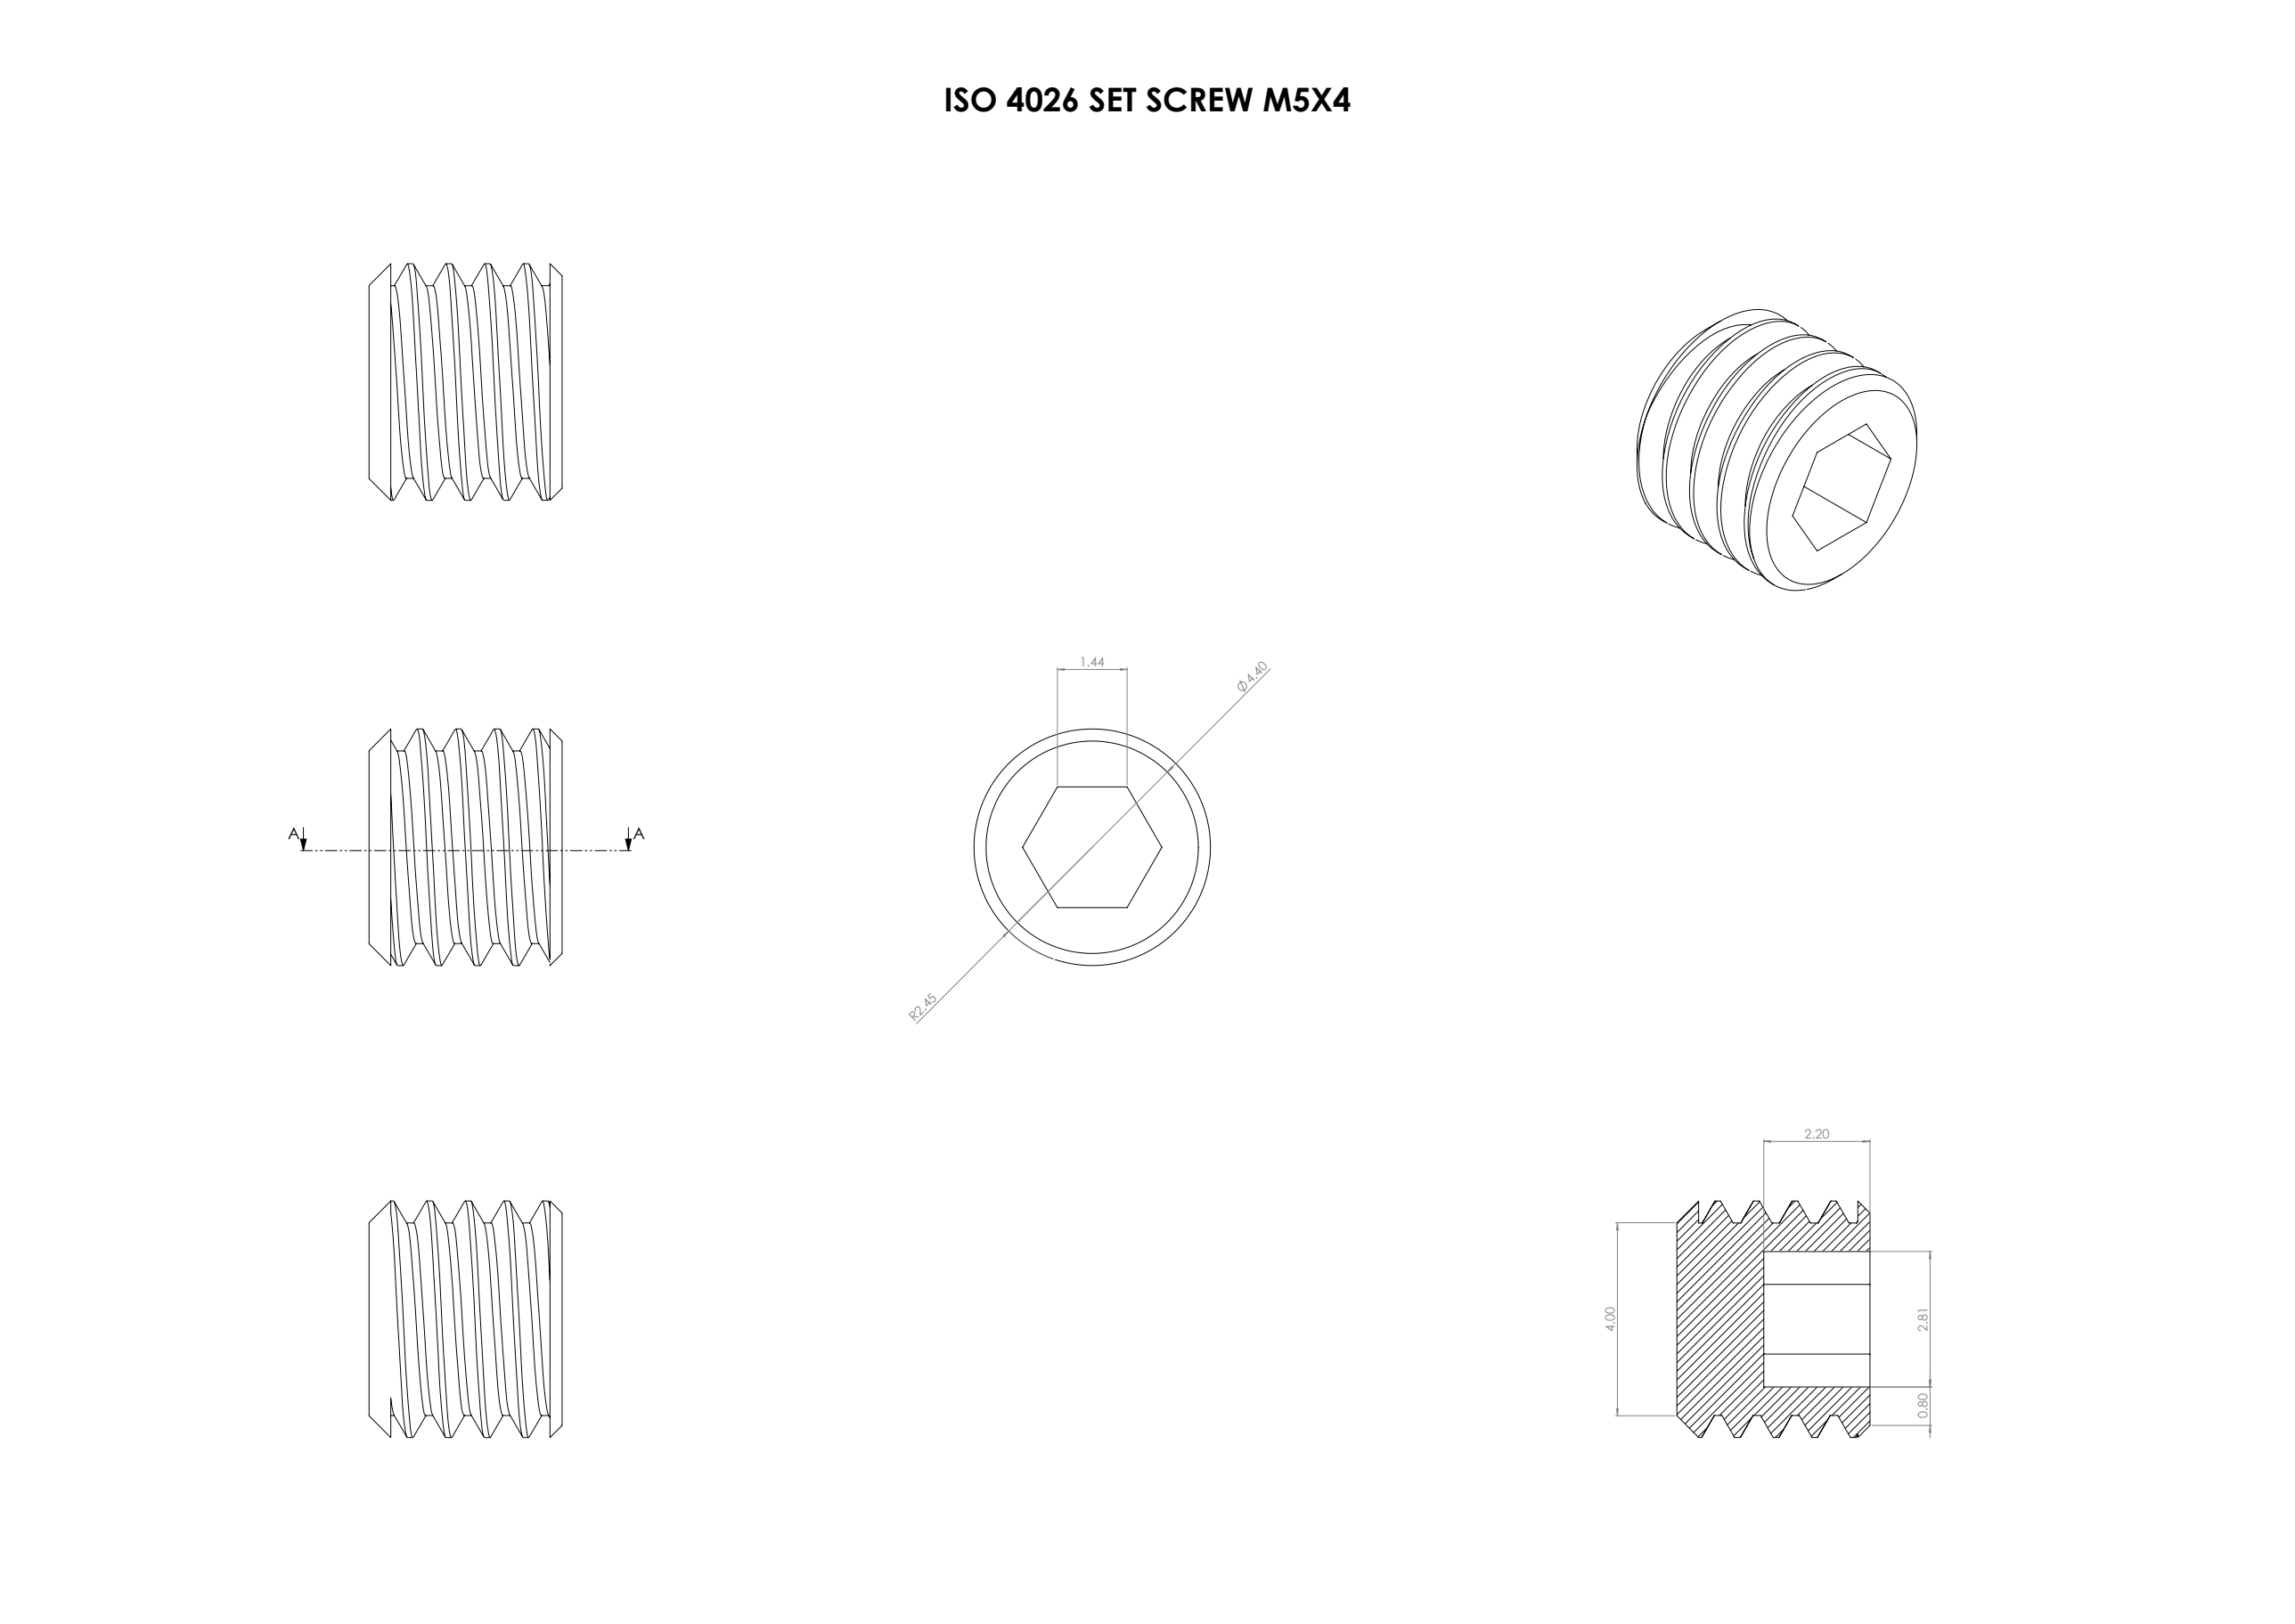
ISO-10303-21;
HEADER;
/* Generated by software containing ST-Developer
 * from STEP Tools, Inc. (www.steptools.com) 
 */

FILE_DESCRIPTION(
/* description */ (''),
/* implementation_level */ '2;1');

FILE_NAME(
/* name */ '11_ISO_4026_Set_Screw_M5x4.step',
/* time_stamp */ '2026-10-21T02:03:06-07:00',
/* author */ (''),
/* organization */ (''),
/* preprocessor_version */ 'ST-DEVELOPER v20.2',
/* originating_system */ 'Autodesk Translation Framework v15.15.0.0',
/* authorisation */ '');

FILE_SCHEMA (('AUTOMOTIVE_DESIGN { 1 0 10303 214 3 1 1 }'));
ENDSEC;

DATA;
#10=MECHANICAL_DESIGN_GEOMETRIC_PRESENTATION_REPRESENTATION('',(#125),#38528);
#87=B_SPLINE_SURFACE_WITH_KNOTS('',3,3,((#35032,#35033,#35034,#35035,#35036,
#35037,#35038,#35039,#35040,#35041,#35042,#35043,#35044,#35045,#35046,#35047,
#35048,#35049,#35050,#35051,#35052,#35053,#35054,#35055,#35056,#35057,#35058,
#35059,#35060,#35061,#35062),(#35063,#35064,#35065,#35066,#35067,#35068,
#35069,#35070,#35071,#35072,#35073,#35074,#35075,#35076,#35077,#35078,#35079,
#35080,#35081,#35082,#35083,#35084,#35085,#35086,#35087,#35088,#35089,#35090,
#35091,#35092,#35093),(#35094,#35095,#35096,#35097,#35098,#35099,#35100,
#35101,#35102,#35103,#35104,#35105,#35106,#35107,#35108,#35109,#35110,#35111,
#35112,#35113,#35114,#35115,#35116,#35117,#35118,#35119,#35120,#35121,#35122,
#35123,#35124),(#35125,#35126,#35127,#35128,#35129,#35130,#35131,#35132,
#35133,#35134,#35135,#35136,#35137,#35138,#35139,#35140,#35141,#35142,#35143,
#35144,#35145,#35146,#35147,#35148,#35149,#35150,#35151,#35152,#35153,#35154,
#35155)),.UNSPECIFIED.,.F.,.F.,.F.,(4,4),(4,1,1,1,1,1,1,1,1,1,1,1,1,1,1,
1,1,1,1,1,1,1,1,1,1,1,1,1,4),(0.,0.0526254770366344),(8.30815772716268,
9.30733212220219,10.3065065172417,11.3056809122812,12.3048553073207,13.3040297023602,
14.3032040973997,15.3023784924392,16.3015528874787,17.3007272825182,18.2999016775577,
19.2990760725973,20.2982504676368,21.2974248626763,22.2965992577158,23.2957736527553,
24.2949480477948,25.2941224428343,26.2932968378738,27.2924712329133,28.2916456279528,
29.2908200229923,30.2899944180318,31.2891688130713,32.2883432081108,33.2875176031503,
34.2866919981899,35.2858663932294,36.2850407882689),.UNSPECIFIED.);
#88=B_SPLINE_SURFACE_WITH_KNOTS('',3,3,((#35379,#35380,#35381,#35382,#35383,
#35384,#35385,#35386,#35387,#35388,#35389,#35390,#35391,#35392,#35393,#35394,
#35395,#35396,#35397,#35398,#35399,#35400,#35401,#35402,#35403,#35404,#35405,
#35406,#35407,#35408,#35409),(#35410,#35411,#35412,#35413,#35414,#35415,
#35416,#35417,#35418,#35419,#35420,#35421,#35422,#35423,#35424,#35425,#35426,
#35427,#35428,#35429,#35430,#35431,#35432,#35433,#35434,#35435,#35436,#35437,
#35438,#35439,#35440),(#35441,#35442,#35443,#35444,#35445,#35446,#35447,
#35448,#35449,#35450,#35451,#35452,#35453,#35454,#35455,#35456,#35457,#35458,
#35459,#35460,#35461,#35462,#35463,#35464,#35465,#35466,#35467,#35468,#35469,
#35470,#35471),(#35472,#35473,#35474,#35475,#35476,#35477,#35478,#35479,
#35480,#35481,#35482,#35483,#35484,#35485,#35486,#35487,#35488,#35489,#35490,
#35491,#35492,#35493,#35494,#35495,#35496,#35497,#35498,#35499,#35500,#35501,
#35502)),.UNSPECIFIED.,.F.,.F.,.F.,(4,4),(4,1,1,1,1,1,1,1,1,1,1,1,1,1,1,
1,1,1,1,1,1,1,1,1,1,1,1,1,4),(0.,0.0526254770366344),(11.6163931973415,
12.615567592381,13.6147419874205,14.61391638246,15.6130907774995,16.612265172539,
17.6114395675785,18.610613962618,19.6097883576575,20.6089627526971,21.6081371477366,
22.6073115427761,23.6064859378156,24.6056603328551,25.6048347278946,26.6040091229341,
27.6031835179736,28.6023579130131,29.6015323080526,30.6007067030921,31.5998810981316,
32.5990554931711,33.5982298882106,34.5974042832501,35.5965786782897,36.5957530733292,
37.5949274683687,38.5941018634082,39.5932762584477),.UNSPECIFIED.);
#101=SHAPE_REPRESENTATION_RELATIONSHIP('SRR','None',#38586,#113);
#113=ADVANCED_BREP_SHAPE_REPRESENTATION('',(#137),#38526);
#125=STYLED_ITEM('',(#38713),#137);
#137=MANIFOLD_SOLID_BREP('Body1',#17082);
#386=CYLINDRICAL_SURFACE('',#18775,2.4505);
#387=CYLINDRICAL_SURFACE('',#18777,2.4505);
#388=CYLINDRICAL_SURFACE('',#18778,2.4505);
#389=CYLINDRICAL_SURFACE('',#18779,2.4505);
#390=CYLINDRICAL_SURFACE('',#18780,1.99475);
#391=CYLINDRICAL_SURFACE('',#18782,1.99475);
#392=CYLINDRICAL_SURFACE('',#18783,1.99475);
#393=CYLINDRICAL_SURFACE('',#18784,1.99475);
#394=CYLINDRICAL_SURFACE('',#18792,1.99475);
#395=CYLINDRICAL_SURFACE('',#18803,2.4505);
#757=B_SPLINE_CURVE_WITH_KNOTS('',3,(#34595,#34596,#34597,#34598,#34599,
#34600,#34601,#34602,#34603,#34604),.UNSPECIFIED.,.F.,.F.,(4,3,3,4),(-4.09157007060746,
-3.99669758015803,-2.99752318511852,-2.06659765062436),.UNSPECIFIED.);
#758=B_SPLINE_CURVE_WITH_KNOTS('',3,(#34607,#34608,#34609,#34610,#34611,
#34612,#34613),.UNSPECIFIED.,.F.,.F.,(4,3,4),(0.,0.999174395039508,1.11662023360669),
 .UNSPECIFIED.);
#759=B_SPLINE_CURVE_WITH_KNOTS('',3,(#34618,#34619,#34620,#34621,#34622,
#34623,#34624,#34625,#34626,#34627,#34628,#34629,#34630,#34631,#34632,#34633,
#34634,#34635,#34636,#34637,#34638,#34639),.UNSPECIFIED.,.F.,.F.,(4,3,3,
3,3,3,3,4),(-10.3747553777871,-9.99174395039507,-8.99256955535556,-7.99339516031606,
-6.99422076527655,-5.99504637023704,-4.99587197519754,-4.09157007060746),
 .UNSPECIFIED.);
#760=B_SPLINE_CURVE_WITH_KNOTS('',3,(#34640,#34641,#34642,#34643,#34644,
#34645,#34646,#34647,#34648,#34649,#34650,#34651,#34652,#34653,#34654,#34655,
#34656,#34657,#34658,#34659,#34660,#34661),.UNSPECIFIED.,.F.,.F.,(4,3,3,
3,3,3,3,4),(1.11662023360669,1.99834879007901,2.99752318511852,3.99669758015803,
4.99587197519753,5.99504637023704,6.99422076527654,7.39980554078627),
 .UNSPECIFIED.);
#761=B_SPLINE_CURVE_WITH_KNOTS('',3,(#34666,#34667,#34668,#34669,#34670,
#34671,#34672,#34673,#34674,#34675,#34676,#34677,#34678,#34679,#34680,#34681,
#34682,#34683,#34684,#34685,#34686,#34687),.UNSPECIFIED.,.F.,.F.,(4,3,3,
3,3,3,3,4),(-16.6579406849666,-15.9867903206321,-14.9876159255926,-13.9884415305531,
-12.9892671355136,-11.9900927404741,-10.9909183454346,-10.3747553777871),
 .UNSPECIFIED.);
#762=B_SPLINE_CURVE_WITH_KNOTS('',3,(#34688,#34689,#34690,#34691,#34692,
#34693,#34694,#34695,#34696,#34697,#34698,#34699,#34700,#34701,#34702,#34703,
#34704,#34705,#34706,#34707,#34708,#34709),.UNSPECIFIED.,.F.,.F.,(4,3,3,
3,3,3,3,4),(7.39980554078627,7.99339516031605,8.99256955535556,9.99174395039507,
10.9909183454346,11.9900927404741,12.9892671355136,13.6829908479659),
 .UNSPECIFIED.);
#763=B_SPLINE_CURVE_WITH_KNOTS('',3,(#34714,#34715,#34716,#34717,#34718,
#34719,#34720,#34721,#34722,#34723,#34724,#34725,#34726,#34727,#34728,#34729,
#34730,#34731,#34732,#34733,#34734,#34735),.UNSPECIFIED.,.F.,.F.,(4,3,3,
3,3,3,3,4),(-22.9411259921462,-21.9818366908691,-20.9826622958296,-19.9834879007901,
-18.9843135057506,-17.9851391107111,-16.9859647156716,-16.6579406849666),
 .UNSPECIFIED.);
#764=B_SPLINE_CURVE_WITH_KNOTS('',3,(#34736,#34737,#34738,#34739,#34740,
#34741,#34742,#34743,#34744,#34745,#34746,#34747,#34748,#34749,#34750,#34751,
#34752,#34753,#34754,#34755,#34756,#34757),.UNSPECIFIED.,.F.,.F.,(4,3,3,
3,3,3,3,4),(13.6829908479659,13.9884415305531,14.9876159255926,15.9867903206321,
16.9859647156716,17.9851391107111,18.9843135057506,19.9661761551454),
 .UNSPECIFIED.);
#765=B_SPLINE_CURVE_WITH_KNOTS('',3,(#34763,#34764,#34765,#34766,#34767,
#34768,#34769),.UNSPECIFIED.,.F.,.F.,(4,1,1,1,4),(34.5575191894877,34.5974042832501,
35.5965786782897,36.5957530733292,37.5266786078233),.UNSPECIFIED.);
#766=B_SPLINE_CURVE_WITH_KNOTS('',3,(#34772,#34773,#34774,#34775,#34776),
 .UNSPECIFIED.,.F.,.F.,(4,1,4),(34.5575191894877,35.2858663932294,36.2850407882689),
 .UNSPECIFIED.);
#767=B_SPLINE_CURVE_WITH_KNOTS('',3,(#34781,#34782,#34783,#34784,#34785,
#34786,#34787,#34788,#34789,#34790),.UNSPECIFIED.,.F.,.F.,(4,1,1,1,1,1,
1,4),(28.2743338823081,28.6023579130131,29.6015323080526,30.6007067030921,
31.5998810981316,32.5990554931711,33.5982298882106,34.5575191894877),
 .UNSPECIFIED.);
#768=B_SPLINE_CURVE_WITH_KNOTS('',3,(#34791,#34792,#34793,#34794,#34795,
#34796,#34797,#34798,#34799,#34800,#34801),.UNSPECIFIED.,.F.,.F.,(4,1,1,
1,1,1,1,1,4),(28.2743338823081,28.2916456279528,29.2908200229923,30.2899944180318,
31.2891688130713,32.2883432081108,33.2875176031503,34.2866919981899,34.5575191894877),
 .UNSPECIFIED.);
#769=B_SPLINE_CURVE_WITH_KNOTS('',3,(#34806,#34807,#34808,#34809,#34810,
#34811,#34812,#34813,#34814,#34815),.UNSPECIFIED.,.F.,.F.,(4,1,1,1,1,1,
1,4),(21.9911485751285,22.6073115427761,23.6064859378156,24.6056603328551,
25.6048347278946,26.6040091229341,27.6031835179736,28.2743338823081),
 .UNSPECIFIED.);
#770=B_SPLINE_CURVE_WITH_KNOTS('',3,(#34816,#34817,#34818,#34819,#34820,
#34821,#34822,#34823,#34824,#34825),.UNSPECIFIED.,.F.,.F.,(4,1,1,1,1,1,
1,4),(21.9911485751285,22.2965992577158,23.2957736527553,24.2949480477948,
25.2941224428343,26.2932968378738,27.2924712329133,28.2743338823081),
 .UNSPECIFIED.);
#771=B_SPLINE_CURVE_WITH_KNOTS('',3,(#34830,#34831,#34832,#34833,#34834,
#34835,#34836,#34837,#34838,#34839),.UNSPECIFIED.,.F.,.F.,(4,1,1,1,1,1,
1,4),(15.707963267949,16.612265172539,17.6114395675785,18.610613962618,
19.6097883576575,20.6089627526971,21.6081371477366,21.9911485751285),
 .UNSPECIFIED.);
#772=B_SPLINE_CURVE_WITH_KNOTS('',3,(#34840,#34841,#34842,#34843,#34844,
#34845,#34846,#34847,#34848,#34849),.UNSPECIFIED.,.F.,.F.,(4,1,1,1,1,1,
1,4),(15.707963267949,16.3015528874787,17.3007272825182,18.2999016775577,
19.2990760725973,20.2982504676368,21.2974248626763,21.9911485751285),
 .UNSPECIFIED.);
#773=B_SPLINE_CURVE_WITH_KNOTS('',3,(#34852,#34853,#34854,#34855,#34856,
#34857,#34858,#34859,#34860,#34861,#34862,#34863,#34864,#34865,#34866,#34867,
#34868,#34869,#34870,#34871,#34872,#34873,#34874,#34875,#34876,#34877,#34878,
#34879,#34880,#34881,#34882,#34883,#34884,#34885,#34886,#34887,#34888,#34889,
#34890,#34891,#34892,#34893,#34894,#34895,#34896,#34897,#34898,#34899,#34900,
#34901,#34902,#34903,#34904,#34905,#34906,#34907,#34908,#34909,#34910,#34911,
#34912,#34913,#34914,#34915,#34916,#34917,#34918,#34919,#34920,#34921,#34922,
#34923,#34924,#34925,#34926,#34927,#34928,#34929,#34930,#34931,#34932,#34933,
#34934,#34935,#34936,#34937,#34938,#34939),.UNSPECIFIED.,.F.,.F.,(4,3,3,
3,3,3,3,3,3,3,3,3,3,3,3,3,3,3,3,3,3,3,3,3,3,3,3,3,3,4),(-0.463803050843695,
-0.449990761124198,-0.428296524385296,-0.416270113415759,-0.41034182721078,
-0.406031993683804,-0.383353142504459,-0.364918243300489,-0.357623436893478,
-0.352445440792161,-0.329117850494041,-0.305348418252453,-0.287979800907514,
-0.27495333789881,-0.271003592095896,-0.246574718000476,-0.235873948872699,
-0.212294861299806,-0.188221669997877,-0.184247659311273,-0.180472049728776,
-0.156013909098849,-0.131078945975368,-0.105968578777427,-0.0960005902951454,
-0.0910052533817002,-0.0652636023140419,-0.03948256399711,-0.0142485222596106,
0.),.UNSPECIFIED.);
#774=B_SPLINE_CURVE_WITH_KNOTS('',3,(#34944,#34945,#34946,#34947,#34948,
#34949,#34950,#34951,#34952,#34953,#34954,#34955,#34956,#34957,#34958,#34959,
#34960,#34961,#34962,#34963,#34964,#34965,#34966,#34967,#34968,#34969,#34970,
#34971,#34972,#34973,#34974,#34975,#34976,#34977,#34978,#34979,#34980,#34981,
#34982,#34983,#34984,#34985,#34986,#34987,#34988,#34989,#34990,#34991,#34992,
#34993,#34994,#34995,#34996,#34997,#34998,#34999,#35000,#35001,#35002,#35003,
#35004,#35005,#35006,#35007,#35008,#35009,#35010,#35011,#35012,#35013,#35014,
#35015,#35016,#35017,#35018,#35019,#35020,#35021,#35022,#35023,#35024,#35025,
#35026,#35027,#35028,#35029,#35030,#35031),.UNSPECIFIED.,.F.,.F.,(4,3,3,
3,3,3,3,3,3,3,3,3,3,3,3,3,3,3,3,3,3,3,3,3,3,3,3,3,3,4),(-0.46178896489977,
-0.445096409523187,-0.41948010739612,-0.406506945826406,-0.398412550454382,
-0.393270804127913,-0.367882741380425,-0.348386088992959,-0.338710078205615,
-0.332907547801024,-0.308142244019199,-0.283899773513071,-0.26018963968495,
-0.251870459427571,-0.247081329031836,-0.243331119007966,-0.219855106139638,
-0.211909522280695,-0.187951737144655,-0.164457770001573,-0.15868347025795,
-0.135324913286723,-0.111987831540051,-0.0890431146252489,-0.0803312568299254,
-0.0766174929132729,-0.0541552161857382,-0.0320577725876878,-0.0106683587118627,
0.),.UNSPECIFIED.);
#775=B_SPLINE_CURVE_WITH_KNOTS('',3,(#35156,#35157,#35158,#35159,#35160,
#35161,#35162,#35163,#35164,#35165,#35166,#35167,#35168,#35169,#35170,#35171,
#35172,#35173,#35174,#35175,#35176,#35177),.UNSPECIFIED.,.F.,.F.,(4,3,3,
3,3,3,3,4),(19.9661761551454,19.9834879007901,20.9826622958296,21.9818366908691,
22.9810110859087,23.9801854809482,24.9793598759877,25.9102854104818),
 .UNSPECIFIED.);
#776=B_SPLINE_CURVE_WITH_KNOTS('',3,(#35179,#35180,#35181,#35182,#35183,
#35184,#35185,#35186,#35187,#35188,#35189,#35190,#35191,#35192,#35193,#35194,
#35195,#35196,#35197,#35198,#35199,#35200,#35201,#35202,#35203,#35204,#35205,
#35206,#35207,#35208,#35209,#35210,#35211,#35212,#35213,#35214,#35215,#35216,
#35217,#35218,#35219,#35220,#35221,#35222,#35223,#35224,#35225,#35226,#35227,
#35228,#35229,#35230,#35231,#35232,#35233,#35234,#35235,#35236,#35237,#35238,
#35239,#35240,#35241,#35242,#35243,#35244,#35245,#35246,#35247,#35248,#35249,
#35250,#35251,#35252,#35253,#35254,#35255,#35256,#35257,#35258,#35259,#35260,
#35261,#35262,#35263,#35264,#35265,#35266),.UNSPECIFIED.,.F.,.F.,(4,3,3,
3,3,3,3,3,3,3,3,3,3,3,3,3,3,3,3,3,3,3,3,3,3,3,3,3,3,4),(-0.463803050843709,
-0.449990761124214,-0.428296490111524,-0.416270081284097,-0.410341690806036,
-0.406031962003142,-0.383353089621238,-0.364918197027671,-0.357623306842884,
-0.35244540774759,-0.329117799946646,-0.305348369315656,-0.287979764204916,
-0.274953310371862,-0.271003565635767,-0.246574693089584,-0.235873948872699,
-0.21229484773092,-0.188221640039157,-0.184247642913191,-0.180472048117772,
-0.15601389132531,-0.131078912920519,-0.105968544178087,-0.096000611432122,
-0.0910052576643347,-0.0652635971708748,-0.0394825672375708,-0.014248568646013,
0.),.UNSPECIFIED.);
#777=B_SPLINE_CURVE_WITH_KNOTS('',3,(#35267,#35268,#35269,#35270,#35271,
#35272,#35273,#35274,#35275),.UNSPECIFIED.,.F.,.F.,(4,1,1,1,1,1,4),(10.374755377787,
11.3056809122812,12.3048553073207,13.3040297023602,14.3032040973997,15.3023784924392,
15.707963267949),.UNSPECIFIED.);
#778=B_SPLINE_CURVE_WITH_KNOTS('',3,(#35281,#35282,#35283,#35284,#35285,
#35286,#35287,#35288,#35289,#35290,#35291,#35292,#35293,#35294,#35295,#35296,
#35297,#35298,#35299,#35300,#35301,#35302,#35303,#35304,#35305,#35306,#35307,
#35308,#35309,#35310,#35311,#35312,#35313,#35314,#35315,#35316,#35317,#35318,
#35319,#35320,#35321,#35322,#35323,#35324,#35325,#35326,#35327,#35328,#35329,
#35330,#35331,#35332,#35333,#35334,#35335,#35336,#35337,#35338,#35339,#35340,
#35341,#35342,#35343,#35344,#35345,#35346,#35347,#35348,#35349,#35350,#35351,
#35352,#35353,#35354,#35355,#35356,#35357,#35358,#35359,#35360,#35361,#35362,
#35363,#35364,#35365,#35366,#35367,#35368),.UNSPECIFIED.,.F.,.F.,(4,3,3,
3,3,3,3,3,3,3,3,3,3,3,3,3,3,3,3,3,3,3,3,3,3,3,3,3,3,4),(-0.461788964899768,
-0.445096409523188,-0.419480109352795,-0.406506947660789,-0.398412571668129,
-0.393270813953603,-0.367882751783358,-0.348386098095525,-0.338710098423989,
-0.332907549361998,-0.308142248257406,-0.283899804164729,-0.260189710156508,
-0.251870630384198,-0.247081550599562,-0.243331158606442,-0.219855173637982,
-0.211909522280694,-0.187951756384898,-0.164457786836786,-0.158683460701996,
-0.135324913663822,-0.111987815902327,-0.0890430596778552,-0.0803312466615788,
-0.0766174883386559,-0.0541551823514923,-0.0320576942341872,-0.0106682241746107,
0.),.UNSPECIFIED.);
#779=B_SPLINE_CURVE_WITH_KNOTS('',3,(#35371,#35372,#35373,#35374,#35375,
#35376,#35377,#35378),.UNSPECIFIED.,.F.,.F.,(4,1,1,1,1,4),(11.6163931973415,
12.615567592381,13.6147419874205,14.61391638246,15.6130907774995,15.707963267949),
 .UNSPECIFIED.);
#780=B_SPLINE_CURVE_WITH_KNOTS('',3,(#35503,#35504,#35505,#35506,#35507,
#35508,#35509,#35510,#35511,#35512,#35513,#35514,#35515,#35516,#35517,#35518,
#35519,#35520,#35521),.UNSPECIFIED.,.F.,.F.,(4,3,3,3,3,3,4),(-27.9768830611062,
-26.9777086660667,-25.9785342710272,-24.9793598759877,-23.9801854809482,
-22.9810110859087,-22.9411259921462),.UNSPECIFIED.);
#1046=CONICAL_SURFACE('',#18802,2.25,0.785398163397448);
#1047=CONICAL_SURFACE('',#18805,2.35,0.785398163397447);
#1475=FACE_BOUND('',#4158,.T.);
#2199=CIRCLE('',#18776,2.4505);
#2200=CIRCLE('',#18781,1.99475);
#2201=CIRCLE('',#18786,2.4505);
#2202=CIRCLE('',#18787,2.4505);
#2203=CIRCLE('',#18789,2.4505);
#2204=CIRCLE('',#18790,2.4505);
#2205=CIRCLE('',#18791,1.99475);
#2206=CIRCLE('',#18801,2.);
#2207=CIRCLE('',#18804,2.4505);
#2208=CIRCLE('',#18806,2.2);
#3107=FACE_OUTER_BOUND('',#4133,.T.);
#3108=FACE_OUTER_BOUND('',#4134,.T.);
#3109=FACE_OUTER_BOUND('',#4135,.T.);
#3110=FACE_OUTER_BOUND('',#4136,.T.);
#3111=FACE_OUTER_BOUND('',#4137,.T.);
#3112=FACE_OUTER_BOUND('',#4138,.T.);
#3113=FACE_OUTER_BOUND('',#4139,.T.);
#3114=FACE_OUTER_BOUND('',#4140,.T.);
#3115=FACE_OUTER_BOUND('',#4141,.T.);
#3116=FACE_OUTER_BOUND('',#4142,.T.);
#3117=FACE_OUTER_BOUND('',#4143,.T.);
#3118=FACE_OUTER_BOUND('',#4144,.T.);
#3119=FACE_OUTER_BOUND('',#4145,.T.);
#3120=FACE_OUTER_BOUND('',#4146,.T.);
#3121=FACE_OUTER_BOUND('',#4147,.T.);
#3122=FACE_OUTER_BOUND('',#4148,.T.);
#3123=FACE_OUTER_BOUND('',#4149,.T.);
#3124=FACE_OUTER_BOUND('',#4150,.T.);
#3125=FACE_OUTER_BOUND('',#4151,.T.);
#3126=FACE_OUTER_BOUND('',#4152,.T.);
#3127=FACE_OUTER_BOUND('',#4153,.T.);
#3128=FACE_OUTER_BOUND('',#4154,.T.);
#3129=FACE_OUTER_BOUND('',#4155,.T.);
#3130=FACE_OUTER_BOUND('',#4156,.T.);
#3131=FACE_OUTER_BOUND('',#4157,.T.);
#4133=EDGE_LOOP('',(#14731,#14732,#14733,#14734));
#4134=EDGE_LOOP('',(#14735,#14736,#14737,#14738));
#4135=EDGE_LOOP('',(#14739,#14740,#14741,#14742));
#4136=EDGE_LOOP('',(#14743,#14744,#14745,#14746));
#4137=EDGE_LOOP('',(#14747,#14748,#14749,#14750));
#4138=EDGE_LOOP('',(#14751,#14752,#14753,#14754));
#4139=EDGE_LOOP('',(#14755,#14756,#14757,#14758));
#4140=EDGE_LOOP('',(#14759,#14760,#14761,#14762));
#4141=EDGE_LOOP('',(#14763,#14764,#14765,#14766,#14767));
#4142=EDGE_LOOP('',(#14768,#14769,#14770,#14771,#14772,#14773,#14774,#14775,
#14776,#14777,#14778,#14779));
#4143=EDGE_LOOP('',(#14780,#14781,#14782,#14783,#14784));
#4144=EDGE_LOOP('',(#14785,#14786,#14787,#14788));
#4145=EDGE_LOOP('',(#14789,#14790,#14791,#14792,#14793,#14794,#14795,#14796,
#14797,#14798,#14799,#14800));
#4146=EDGE_LOOP('',(#14801,#14802,#14803,#14804));
#4147=EDGE_LOOP('',(#14805,#14806,#14807,#14808));
#4148=EDGE_LOOP('',(#14809,#14810,#14811,#14812));
#4149=EDGE_LOOP('',(#14813,#14814,#14815,#14816));
#4150=EDGE_LOOP('',(#14817,#14818,#14819,#14820));
#4151=EDGE_LOOP('',(#14821,#14822,#14823,#14824));
#4152=EDGE_LOOP('',(#14825,#14826,#14827,#14828,#14829,#14830));
#4153=EDGE_LOOP('',(#14831));
#4154=EDGE_LOOP('',(#14832,#14833,#14834,#14835,#14836,#14837));
#4155=EDGE_LOOP('',(#14838,#14839,#14840,#14841));
#4156=EDGE_LOOP('',(#14842,#14843,#14844,#14845,#14846,#14847));
#4157=EDGE_LOOP('',(#14848));
#4158=EDGE_LOOP('',(#14849,#14850,#14851,#14852,#14853,#14854));
#5055=LINE('',#34593,#6030);
#5056=LINE('',#34617,#6031);
#5057=LINE('',#34665,#6032);
#5058=LINE('',#34713,#6033);
#5059=LINE('',#34761,#6034);
#5060=LINE('',#34780,#6035);
#5061=LINE('',#34805,#6036);
#5062=LINE('',#34829,#6037);
#5063=LINE('',#35525,#6038);
#5064=LINE('',#35527,#6039);
#5065=LINE('',#35529,#6040);
#5066=LINE('',#35530,#6041);
#5067=LINE('',#35533,#6042);
#5068=LINE('',#35535,#6043);
#5069=LINE('',#35536,#6044);
#5070=LINE('',#35539,#6045);
#5071=LINE('',#35541,#6046);
#5072=LINE('',#35542,#6047);
#5073=LINE('',#35545,#6048);
#5074=LINE('',#35547,#6049);
#5075=LINE('',#35548,#6050);
#5076=LINE('',#35551,#6051);
#5077=LINE('',#35553,#6052);
#5078=LINE('',#35554,#6053);
#5079=LINE('',#35556,#6054);
#5080=LINE('',#35557,#6055);
#5081=LINE('',#35563,#6056);
#5082=LINE('',#35569,#6057);
#6030=VECTOR('',#22907,2.5);
#6031=VECTOR('',#22912,2.5);
#6032=VECTOR('',#22915,2.5);
#6033=VECTOR('',#22918,2.5);
#6034=VECTOR('',#22921,1.99475);
#6035=VECTOR('',#22926,1.99475);
#6036=VECTOR('',#22929,1.99475);
#6037=VECTOR('',#22932,1.99475);
#6038=VECTOR('',#22951,10.);
#6039=VECTOR('',#22952,10.);
#6040=VECTOR('',#22953,10.);
#6041=VECTOR('',#22954,10.);
#6042=VECTOR('',#22957,10.);
#6043=VECTOR('',#22958,10.);
#6044=VECTOR('',#22959,10.);
#6045=VECTOR('',#22962,10.);
#6046=VECTOR('',#22963,10.);
#6047=VECTOR('',#22964,10.);
#6048=VECTOR('',#22967,10.);
#6049=VECTOR('',#22968,10.);
#6050=VECTOR('',#22969,10.);
#6051=VECTOR('',#22972,10.);
#6052=VECTOR('',#22973,10.);
#6053=VECTOR('',#22974,10.);
#6054=VECTOR('',#22977,10.);
#6055=VECTOR('',#22978,10.);
#6056=VECTOR('',#22987,2.25);
#6057=VECTOR('',#22996,2.35);
#7589=VERTEX_POINT('',#34591);
#7590=VERTEX_POINT('',#34592);
#7591=VERTEX_POINT('',#34594);
#7592=VERTEX_POINT('',#34605);
#7593=VERTEX_POINT('',#34615);
#7594=VERTEX_POINT('',#34616);
#7595=VERTEX_POINT('',#34663);
#7596=VERTEX_POINT('',#34664);
#7597=VERTEX_POINT('',#34711);
#7598=VERTEX_POINT('',#34712);
#7599=VERTEX_POINT('',#34759);
#7600=VERTEX_POINT('',#34760);
#7601=VERTEX_POINT('',#34762);
#7602=VERTEX_POINT('',#34770);
#7603=VERTEX_POINT('',#34778);
#7604=VERTEX_POINT('',#34779);
#7605=VERTEX_POINT('',#34803);
#7606=VERTEX_POINT('',#34804);
#7607=VERTEX_POINT('',#34827);
#7608=VERTEX_POINT('',#34828);
#7609=VERTEX_POINT('',#34851);
#7610=VERTEX_POINT('',#34940);
#7611=VERTEX_POINT('',#34942);
#7612=VERTEX_POINT('',#35178);
#7613=VERTEX_POINT('',#35277);
#7614=VERTEX_POINT('',#35280);
#7615=VERTEX_POINT('',#35523);
#7616=VERTEX_POINT('',#35524);
#7617=VERTEX_POINT('',#35526);
#7618=VERTEX_POINT('',#35528);
#7619=VERTEX_POINT('',#35532);
#7620=VERTEX_POINT('',#35534);
#7621=VERTEX_POINT('',#35538);
#7622=VERTEX_POINT('',#35540);
#7623=VERTEX_POINT('',#35544);
#7624=VERTEX_POINT('',#35546);
#7625=VERTEX_POINT('',#35550);
#7626=VERTEX_POINT('',#35552);
#7627=VERTEX_POINT('',#35560);
#7628=VERTEX_POINT('',#35567);
#10017=EDGE_CURVE('',#7589,#7590,#5055,.T.);
#10018=EDGE_CURVE('',#7589,#7591,#757,.T.);
#10019=EDGE_CURVE('',#7591,#7592,#2199,.T.);
#10020=EDGE_CURVE('',#7592,#7590,#758,.T.);
#10021=EDGE_CURVE('',#7593,#7594,#5056,.T.);
#10022=EDGE_CURVE('',#7593,#7589,#759,.T.);
#10023=EDGE_CURVE('',#7590,#7594,#760,.T.);
#10024=EDGE_CURVE('',#7595,#7596,#5057,.T.);
#10025=EDGE_CURVE('',#7595,#7593,#761,.T.);
#10026=EDGE_CURVE('',#7594,#7596,#762,.T.);
#10027=EDGE_CURVE('',#7597,#7598,#5058,.T.);
#10028=EDGE_CURVE('',#7597,#7595,#763,.T.);
#10029=EDGE_CURVE('',#7596,#7598,#764,.T.);
#10030=EDGE_CURVE('',#7599,#7600,#5059,.T.);
#10031=EDGE_CURVE('',#7599,#7601,#765,.T.);
#10032=EDGE_CURVE('',#7602,#7601,#2200,.T.);
#10033=EDGE_CURVE('',#7600,#7602,#766,.T.);
#10034=EDGE_CURVE('',#7603,#7604,#5060,.T.);
#10035=EDGE_CURVE('',#7603,#7599,#767,.T.);
#10036=EDGE_CURVE('',#7604,#7600,#768,.T.);
#10037=EDGE_CURVE('',#7605,#7606,#5061,.T.);
#10038=EDGE_CURVE('',#7605,#7603,#769,.T.);
#10039=EDGE_CURVE('',#7606,#7604,#770,.T.);
#10040=EDGE_CURVE('',#7607,#7608,#5062,.T.);
#10041=EDGE_CURVE('',#7607,#7605,#771,.T.);
#10042=EDGE_CURVE('',#7608,#7606,#772,.T.);
#10043=EDGE_CURVE('',#7601,#7609,#773,.T.);
#10044=EDGE_CURVE('',#7610,#7609,#2201,.F.);
#10045=EDGE_CURVE('',#7611,#7610,#2202,.F.);
#10046=EDGE_CURVE('',#7611,#7602,#774,.T.);
#10047=EDGE_CURVE('',#7598,#7611,#775,.T.);
#10048=EDGE_CURVE('',#7612,#7592,#776,.T.);
#10049=EDGE_CURVE('',#7612,#7608,#777,.T.);
#10050=EDGE_CURVE('',#7592,#7613,#2203,.T.);
#10051=EDGE_CURVE('',#7613,#7591,#2204,.T.);
#10052=EDGE_CURVE('',#7591,#7614,#778,.T.);
#10053=EDGE_CURVE('',#7614,#7612,#2205,.T.);
#10054=EDGE_CURVE('',#7614,#7607,#779,.T.);
#10055=EDGE_CURVE('',#7609,#7597,#780,.T.);
#10056=EDGE_CURVE('',#7615,#7616,#5063,.T.);
#10057=EDGE_CURVE('',#7615,#7617,#5064,.T.);
#10058=EDGE_CURVE('',#7617,#7618,#5065,.T.);
#10059=EDGE_CURVE('',#7616,#7618,#5066,.T.);
#10060=EDGE_CURVE('',#7619,#7615,#5067,.T.);
#10061=EDGE_CURVE('',#7619,#7620,#5068,.T.);
#10062=EDGE_CURVE('',#7620,#7617,#5069,.T.);
#10063=EDGE_CURVE('',#7621,#7619,#5070,.T.);
#10064=EDGE_CURVE('',#7621,#7622,#5071,.T.);
#10065=EDGE_CURVE('',#7622,#7620,#5072,.T.);
#10066=EDGE_CURVE('',#7623,#7621,#5073,.T.);
#10067=EDGE_CURVE('',#7623,#7624,#5074,.T.);
#10068=EDGE_CURVE('',#7624,#7622,#5075,.T.);
#10069=EDGE_CURVE('',#7625,#7623,#5076,.T.);
#10070=EDGE_CURVE('',#7625,#7626,#5077,.T.);
#10071=EDGE_CURVE('',#7626,#7624,#5078,.T.);
#10072=EDGE_CURVE('',#7616,#7625,#5079,.T.);
#10073=EDGE_CURVE('',#7618,#7626,#5080,.T.);
#10074=EDGE_CURVE('',#7627,#7627,#2206,.T.);
#10075=EDGE_CURVE('',#7613,#7627,#5081,.T.);
#10076=EDGE_CURVE('',#7609,#7611,#2207,.F.);
#10077=EDGE_CURVE('',#7628,#7628,#2208,.T.);
#10078=EDGE_CURVE('',#7628,#7610,#5082,.T.);
#14731=ORIENTED_EDGE('',*,*,#10017,.F.);
#14732=ORIENTED_EDGE('',*,*,#10018,.T.);
#14733=ORIENTED_EDGE('',*,*,#10019,.T.);
#14734=ORIENTED_EDGE('',*,*,#10020,.T.);
#14735=ORIENTED_EDGE('',*,*,#10021,.F.);
#14736=ORIENTED_EDGE('',*,*,#10022,.T.);
#14737=ORIENTED_EDGE('',*,*,#10017,.T.);
#14738=ORIENTED_EDGE('',*,*,#10023,.T.);
#14739=ORIENTED_EDGE('',*,*,#10024,.F.);
#14740=ORIENTED_EDGE('',*,*,#10025,.T.);
#14741=ORIENTED_EDGE('',*,*,#10021,.T.);
#14742=ORIENTED_EDGE('',*,*,#10026,.T.);
#14743=ORIENTED_EDGE('',*,*,#10027,.F.);
#14744=ORIENTED_EDGE('',*,*,#10028,.T.);
#14745=ORIENTED_EDGE('',*,*,#10024,.T.);
#14746=ORIENTED_EDGE('',*,*,#10029,.T.);
#14747=ORIENTED_EDGE('',*,*,#10030,.F.);
#14748=ORIENTED_EDGE('',*,*,#10031,.T.);
#14749=ORIENTED_EDGE('',*,*,#10032,.F.);
#14750=ORIENTED_EDGE('',*,*,#10033,.F.);
#14751=ORIENTED_EDGE('',*,*,#10034,.F.);
#14752=ORIENTED_EDGE('',*,*,#10035,.T.);
#14753=ORIENTED_EDGE('',*,*,#10030,.T.);
#14754=ORIENTED_EDGE('',*,*,#10036,.F.);
#14755=ORIENTED_EDGE('',*,*,#10037,.F.);
#14756=ORIENTED_EDGE('',*,*,#10038,.T.);
#14757=ORIENTED_EDGE('',*,*,#10034,.T.);
#14758=ORIENTED_EDGE('',*,*,#10039,.F.);
#14759=ORIENTED_EDGE('',*,*,#10040,.F.);
#14760=ORIENTED_EDGE('',*,*,#10041,.T.);
#14761=ORIENTED_EDGE('',*,*,#10037,.T.);
#14762=ORIENTED_EDGE('',*,*,#10042,.F.);
#14763=ORIENTED_EDGE('',*,*,#10032,.T.);
#14764=ORIENTED_EDGE('',*,*,#10043,.T.);
#14765=ORIENTED_EDGE('',*,*,#10044,.F.);
#14766=ORIENTED_EDGE('',*,*,#10045,.F.);
#14767=ORIENTED_EDGE('',*,*,#10046,.T.);
#14768=ORIENTED_EDGE('',*,*,#10046,.F.);
#14769=ORIENTED_EDGE('',*,*,#10047,.F.);
#14770=ORIENTED_EDGE('',*,*,#10029,.F.);
#14771=ORIENTED_EDGE('',*,*,#10026,.F.);
#14772=ORIENTED_EDGE('',*,*,#10023,.F.);
#14773=ORIENTED_EDGE('',*,*,#10020,.F.);
#14774=ORIENTED_EDGE('',*,*,#10048,.F.);
#14775=ORIENTED_EDGE('',*,*,#10049,.T.);
#14776=ORIENTED_EDGE('',*,*,#10042,.T.);
#14777=ORIENTED_EDGE('',*,*,#10039,.T.);
#14778=ORIENTED_EDGE('',*,*,#10036,.T.);
#14779=ORIENTED_EDGE('',*,*,#10033,.T.);
#14780=ORIENTED_EDGE('',*,*,#10050,.T.);
#14781=ORIENTED_EDGE('',*,*,#10051,.T.);
#14782=ORIENTED_EDGE('',*,*,#10052,.T.);
#14783=ORIENTED_EDGE('',*,*,#10053,.T.);
#14784=ORIENTED_EDGE('',*,*,#10048,.T.);
#14785=ORIENTED_EDGE('',*,*,#10040,.T.);
#14786=ORIENTED_EDGE('',*,*,#10049,.F.);
#14787=ORIENTED_EDGE('',*,*,#10053,.F.);
#14788=ORIENTED_EDGE('',*,*,#10054,.T.);
#14789=ORIENTED_EDGE('',*,*,#10043,.F.);
#14790=ORIENTED_EDGE('',*,*,#10031,.F.);
#14791=ORIENTED_EDGE('',*,*,#10035,.F.);
#14792=ORIENTED_EDGE('',*,*,#10038,.F.);
#14793=ORIENTED_EDGE('',*,*,#10041,.F.);
#14794=ORIENTED_EDGE('',*,*,#10054,.F.);
#14795=ORIENTED_EDGE('',*,*,#10052,.F.);
#14796=ORIENTED_EDGE('',*,*,#10018,.F.);
#14797=ORIENTED_EDGE('',*,*,#10022,.F.);
#14798=ORIENTED_EDGE('',*,*,#10025,.F.);
#14799=ORIENTED_EDGE('',*,*,#10028,.F.);
#14800=ORIENTED_EDGE('',*,*,#10055,.F.);
#14801=ORIENTED_EDGE('',*,*,#10056,.F.);
#14802=ORIENTED_EDGE('',*,*,#10057,.T.);
#14803=ORIENTED_EDGE('',*,*,#10058,.T.);
#14804=ORIENTED_EDGE('',*,*,#10059,.F.);
#14805=ORIENTED_EDGE('',*,*,#10060,.F.);
#14806=ORIENTED_EDGE('',*,*,#10061,.T.);
#14807=ORIENTED_EDGE('',*,*,#10062,.T.);
#14808=ORIENTED_EDGE('',*,*,#10057,.F.);
#14809=ORIENTED_EDGE('',*,*,#10063,.F.);
#14810=ORIENTED_EDGE('',*,*,#10064,.T.);
#14811=ORIENTED_EDGE('',*,*,#10065,.T.);
#14812=ORIENTED_EDGE('',*,*,#10061,.F.);
#14813=ORIENTED_EDGE('',*,*,#10066,.F.);
#14814=ORIENTED_EDGE('',*,*,#10067,.T.);
#14815=ORIENTED_EDGE('',*,*,#10068,.T.);
#14816=ORIENTED_EDGE('',*,*,#10064,.F.);
#14817=ORIENTED_EDGE('',*,*,#10069,.F.);
#14818=ORIENTED_EDGE('',*,*,#10070,.T.);
#14819=ORIENTED_EDGE('',*,*,#10071,.T.);
#14820=ORIENTED_EDGE('',*,*,#10067,.F.);
#14821=ORIENTED_EDGE('',*,*,#10072,.F.);
#14822=ORIENTED_EDGE('',*,*,#10059,.T.);
#14823=ORIENTED_EDGE('',*,*,#10073,.T.);
#14824=ORIENTED_EDGE('',*,*,#10070,.F.);
#14825=ORIENTED_EDGE('',*,*,#10073,.F.);
#14826=ORIENTED_EDGE('',*,*,#10058,.F.);
#14827=ORIENTED_EDGE('',*,*,#10062,.F.);
#14828=ORIENTED_EDGE('',*,*,#10065,.F.);
#14829=ORIENTED_EDGE('',*,*,#10068,.F.);
#14830=ORIENTED_EDGE('',*,*,#10071,.F.);
#14831=ORIENTED_EDGE('',*,*,#10074,.F.);
#14832=ORIENTED_EDGE('',*,*,#10050,.F.);
#14833=ORIENTED_EDGE('',*,*,#10019,.F.);
#14834=ORIENTED_EDGE('',*,*,#10051,.F.);
#14835=ORIENTED_EDGE('',*,*,#10075,.T.);
#14836=ORIENTED_EDGE('',*,*,#10074,.T.);
#14837=ORIENTED_EDGE('',*,*,#10075,.F.);
#14838=ORIENTED_EDGE('',*,*,#10027,.T.);
#14839=ORIENTED_EDGE('',*,*,#10047,.T.);
#14840=ORIENTED_EDGE('',*,*,#10076,.F.);
#14841=ORIENTED_EDGE('',*,*,#10055,.T.);
#14842=ORIENTED_EDGE('',*,*,#10077,.F.);
#14843=ORIENTED_EDGE('',*,*,#10078,.T.);
#14844=ORIENTED_EDGE('',*,*,#10044,.T.);
#14845=ORIENTED_EDGE('',*,*,#10076,.T.);
#14846=ORIENTED_EDGE('',*,*,#10045,.T.);
#14847=ORIENTED_EDGE('',*,*,#10078,.F.);
#14848=ORIENTED_EDGE('',*,*,#10077,.T.);
#14849=ORIENTED_EDGE('',*,*,#10056,.T.);
#14850=ORIENTED_EDGE('',*,*,#10072,.T.);
#14851=ORIENTED_EDGE('',*,*,#10069,.T.);
#14852=ORIENTED_EDGE('',*,*,#10066,.T.);
#14853=ORIENTED_EDGE('',*,*,#10063,.T.);
#14854=ORIENTED_EDGE('',*,*,#10060,.T.);
#15984=PLANE('',#18785);
#15985=PLANE('',#18788);
#15986=PLANE('',#18793);
#15987=PLANE('',#18794);
#15988=PLANE('',#18795);
#15989=PLANE('',#18796);
#15990=PLANE('',#18797);
#15991=PLANE('',#18798);
#15992=PLANE('',#18799);
#15993=PLANE('',#18800);
#15994=PLANE('',#18807);
#16916=ADVANCED_FACE('',(#3107),#386,.T.);
#16917=ADVANCED_FACE('',(#3108),#387,.T.);
#16918=ADVANCED_FACE('',(#3109),#388,.T.);
#16919=ADVANCED_FACE('',(#3110),#389,.T.);
#16920=ADVANCED_FACE('',(#3111),#390,.T.);
#16921=ADVANCED_FACE('',(#3112),#391,.T.);
#16922=ADVANCED_FACE('',(#3113),#392,.T.);
#16923=ADVANCED_FACE('',(#3114),#393,.T.);
#16924=ADVANCED_FACE('',(#3115),#15984,.F.);
#16925=ADVANCED_FACE('',(#3116),#87,.F.);
#16926=ADVANCED_FACE('',(#3117),#15985,.T.);
#16927=ADVANCED_FACE('',(#3118),#394,.T.);
#16928=ADVANCED_FACE('',(#3119),#88,.F.);
#16929=ADVANCED_FACE('',(#3120),#15986,.F.);
#16930=ADVANCED_FACE('',(#3121),#15987,.F.);
#16931=ADVANCED_FACE('',(#3122),#15988,.F.);
#16932=ADVANCED_FACE('',(#3123),#15989,.F.);
#16933=ADVANCED_FACE('',(#3124),#15990,.F.);
#16934=ADVANCED_FACE('',(#3125),#15991,.F.);
#16935=ADVANCED_FACE('',(#3126),#15992,.F.);
#16936=ADVANCED_FACE('',(#3127),#15993,.T.);
#16937=ADVANCED_FACE('',(#3128),#1046,.T.);
#16938=ADVANCED_FACE('',(#3129),#395,.T.);
#16939=ADVANCED_FACE('',(#3130),#1047,.T.);
#16940=ADVANCED_FACE('',(#3131,#1475),#15994,.T.);
#17082=CLOSED_SHELL('',(#16916,#16917,#16918,#16919,#16920,#16921,#16922,
#16923,#16924,#16925,#16926,#16927,#16928,#16929,#16930,#16931,#16932,#16933,
#16934,#16935,#16936,#16937,#16938,#16939,#16940));
#18774=AXIS2_PLACEMENT_3D('',#34589,#22903,#22904);
#18775=AXIS2_PLACEMENT_3D('',#34590,#22905,#22906);
#18776=AXIS2_PLACEMENT_3D('',#34606,#22908,#22909);
#18777=AXIS2_PLACEMENT_3D('',#34614,#22910,#22911);
#18778=AXIS2_PLACEMENT_3D('',#34662,#22913,#22914);
#18779=AXIS2_PLACEMENT_3D('',#34710,#22916,#22917);
#18780=AXIS2_PLACEMENT_3D('',#34758,#22919,#22920);
#18781=AXIS2_PLACEMENT_3D('',#34771,#22922,#22923);
#18782=AXIS2_PLACEMENT_3D('',#34777,#22924,#22925);
#18783=AXIS2_PLACEMENT_3D('',#34802,#22927,#22928);
#18784=AXIS2_PLACEMENT_3D('',#34826,#22930,#22931);
#18785=AXIS2_PLACEMENT_3D('',#34850,#22933,#22934);
#18786=AXIS2_PLACEMENT_3D('',#34941,#22935,#22936);
#18787=AXIS2_PLACEMENT_3D('',#34943,#22937,#22938);
#18788=AXIS2_PLACEMENT_3D('',#35276,#22939,#22940);
#18789=AXIS2_PLACEMENT_3D('',#35278,#22941,#22942);
#18790=AXIS2_PLACEMENT_3D('',#35279,#22943,#22944);
#18791=AXIS2_PLACEMENT_3D('',#35369,#22945,#22946);
#18792=AXIS2_PLACEMENT_3D('',#35370,#22947,#22948);
#18793=AXIS2_PLACEMENT_3D('',#35522,#22949,#22950);
#18794=AXIS2_PLACEMENT_3D('',#35531,#22955,#22956);
#18795=AXIS2_PLACEMENT_3D('',#35537,#22960,#22961);
#18796=AXIS2_PLACEMENT_3D('',#35543,#22965,#22966);
#18797=AXIS2_PLACEMENT_3D('',#35549,#22970,#22971);
#18798=AXIS2_PLACEMENT_3D('',#35555,#22975,#22976);
#18799=AXIS2_PLACEMENT_3D('',#35558,#22979,#22980);
#18800=AXIS2_PLACEMENT_3D('',#35559,#22981,#22982);
#18801=AXIS2_PLACEMENT_3D('',#35561,#22983,#22984);
#18802=AXIS2_PLACEMENT_3D('',#35562,#22985,#22986);
#18803=AXIS2_PLACEMENT_3D('',#35564,#22988,#22989);
#18804=AXIS2_PLACEMENT_3D('',#35565,#22990,#22991);
#18805=AXIS2_PLACEMENT_3D('',#35566,#22992,#22993);
#18806=AXIS2_PLACEMENT_3D('',#35568,#22994,#22995);
#18807=AXIS2_PLACEMENT_3D('',#35570,#22997,#22998);
#22903=DIRECTION('axis',(0.,0.,1.));
#22904=DIRECTION('refdir',(1.,0.,0.));
#22905=DIRECTION('center_axis',(1.,0.,0.));
#22906=DIRECTION('ref_axis',(0.,1.,0.));
#22907=DIRECTION('',(-1.,0.,0.));
#22908=DIRECTION('center_axis',(1.,0.,0.));
#22909=DIRECTION('ref_axis',(0.,1.,0.));
#22910=DIRECTION('center_axis',(1.,0.,0.));
#22911=DIRECTION('ref_axis',(0.,1.,0.));
#22912=DIRECTION('',(-1.,0.,0.));
#22913=DIRECTION('center_axis',(1.,0.,0.));
#22914=DIRECTION('ref_axis',(0.,1.,0.));
#22915=DIRECTION('',(-1.,0.,0.));
#22916=DIRECTION('center_axis',(1.,0.,0.));
#22917=DIRECTION('ref_axis',(0.,1.,0.));
#22918=DIRECTION('',(-1.,0.,0.));
#22919=DIRECTION('center_axis',(1.,0.,0.));
#22920=DIRECTION('ref_axis',(6.95715643956108E-17,-0.0863639019455519,-0.996263658094954));
#22921=DIRECTION('',(1.,0.,0.));
#22922=DIRECTION('center_axis',(1.,0.,0.));
#22923=DIRECTION('ref_axis',(6.95715643956108E-17,1.,6.84751808553105E-15));
#22924=DIRECTION('center_axis',(1.,0.,0.));
#22925=DIRECTION('ref_axis',(6.95715643956108E-17,1.,6.84751808553105E-15));
#22926=DIRECTION('',(1.,0.,0.));
#22927=DIRECTION('center_axis',(1.,0.,0.));
#22928=DIRECTION('ref_axis',(6.95715643956108E-17,1.,6.84751808553105E-15));
#22929=DIRECTION('',(1.,0.,0.));
#22930=DIRECTION('center_axis',(1.,0.,0.));
#22931=DIRECTION('ref_axis',(6.95715643956108E-17,1.,6.84751808553105E-15));
#22932=DIRECTION('',(1.,0.,0.));
#22933=DIRECTION('center_axis',(1.,0.,0.));
#22934=DIRECTION('ref_axis',(0.,0.,-1.));
#22935=DIRECTION('center_axis',(-1.,0.,0.));
#22936=DIRECTION('ref_axis',(0.,1.,0.));
#22937=DIRECTION('center_axis',(-1.,0.,0.));
#22938=DIRECTION('ref_axis',(0.,1.,0.));
#22939=DIRECTION('center_axis',(1.,0.,0.));
#22940=DIRECTION('ref_axis',(0.,0.,-1.));
#22941=DIRECTION('center_axis',(1.,0.,0.));
#22942=DIRECTION('ref_axis',(0.,1.,0.));
#22943=DIRECTION('center_axis',(1.,0.,0.));
#22944=DIRECTION('ref_axis',(0.,1.,0.));
#22945=DIRECTION('center_axis',(-1.,0.,0.));
#22946=DIRECTION('ref_axis',(6.95715643956108E-17,1.,6.84751808553105E-15));
#22947=DIRECTION('center_axis',(1.,0.,0.));
#22948=DIRECTION('ref_axis',(6.95715643956108E-17,1.,6.84751808553105E-15));
#22949=DIRECTION('center_axis',(0.,0.5,0.866025403784439));
#22950=DIRECTION('ref_axis',(0.,0.866025403784439,-0.5));
#22951=DIRECTION('',(0.,0.866025403784439,-0.5));
#22952=DIRECTION('',(-1.,0.,0.));
#22953=DIRECTION('',(0.,0.866025403784439,-0.5));
#22954=DIRECTION('',(-1.,0.,0.));
#22955=DIRECTION('center_axis',(0.,-0.5,0.866025403784439));
#22956=DIRECTION('ref_axis',(0.,0.866025403784439,0.5));
#22957=DIRECTION('',(0.,0.866025403784439,0.5));
#22958=DIRECTION('',(-1.,0.,0.));
#22959=DIRECTION('',(0.,0.866025403784439,0.5));
#22960=DIRECTION('center_axis',(0.,-1.,-1.92296268638356E-16));
#22961=DIRECTION('ref_axis',(0.,-1.92296268638356E-16,1.));
#22962=DIRECTION('',(0.,-1.92296268638356E-16,1.));
#22963=DIRECTION('',(-1.,0.,0.));
#22964=DIRECTION('',(0.,-1.92296268638356E-16,1.));
#22965=DIRECTION('center_axis',(0.,-0.5,-0.866025403784439));
#22966=DIRECTION('ref_axis',(0.,-0.866025403784439,0.5));
#22967=DIRECTION('',(0.,-0.866025403784439,0.5));
#22968=DIRECTION('',(-1.,0.,0.));
#22969=DIRECTION('',(0.,-0.866025403784439,0.5));
#22970=DIRECTION('center_axis',(0.,0.5,-0.866025403784439));
#22971=DIRECTION('ref_axis',(0.,-0.866025403784439,-0.5));
#22972=DIRECTION('',(0.,-0.866025403784439,-0.5));
#22973=DIRECTION('',(-1.,0.,0.));
#22974=DIRECTION('',(0.,-0.866025403784439,-0.5));
#22975=DIRECTION('center_axis',(0.,1.,-3.84592537276713E-16));
#22976=DIRECTION('ref_axis',(0.,-3.84592537276713E-16,-1.));
#22977=DIRECTION('',(0.,-3.84592537276713E-16,-1.));
#22978=DIRECTION('',(0.,-3.84592537276713E-16,-1.));
#22979=DIRECTION('center_axis',(-1.,0.,0.));
#22980=DIRECTION('ref_axis',(0.,0.,1.));
#22981=DIRECTION('center_axis',(-1.,0.,0.));
#22982=DIRECTION('ref_axis',(0.,0.,1.));
#22983=DIRECTION('center_axis',(1.,0.,0.));
#22984=DIRECTION('ref_axis',(0.,0.,-1.));
#22985=DIRECTION('center_axis',(1.,0.,0.));
#22986=DIRECTION('ref_axis',(0.,1.,0.));
#22987=DIRECTION('',(-0.707106781186548,0.707106781186547,8.65956056235493E-17));
#22988=DIRECTION('center_axis',(1.,0.,0.));
#22989=DIRECTION('ref_axis',(0.,1.,0.));
#22990=DIRECTION('center_axis',(-1.,0.,0.));
#22991=DIRECTION('ref_axis',(0.,1.,0.));
#22992=DIRECTION('center_axis',(-1.,0.,0.));
#22993=DIRECTION('ref_axis',(0.,1.,0.));
#22994=DIRECTION('center_axis',(1.,0.,0.));
#22995=DIRECTION('ref_axis',(0.,0.,-1.));
#22996=DIRECTION('',(-0.707106781186548,-0.707106781186547,-8.65956056235493E-17));
#22997=DIRECTION('center_axis',(1.,0.,0.));
#22998=DIRECTION('ref_axis',(0.,0.,-1.));
#34589=CARTESIAN_POINT('',(0.,0.,0.));
#34590=CARTESIAN_POINT('Origin',(2.1,0.,0.));
#34591=CARTESIAN_POINT('',(0.708327496212055,-2.45360913320878,0.00150472093799672));
#34592=CARTESIAN_POINT('',(0.592672503787945,-2.45282685237657,0.00258448634202159));
#34593=CARTESIAN_POINT('',(2.1,-2.4505,-3.00099698131059E-16));
#34594=CARTESIAN_POINT('',(0.4505,1.0763748274605,2.20373264345719));
#34595=CARTESIAN_POINT('Ctrl Pts',(0.708327496212055,-2.45360913320878,
0.00150472093799672));
#34596=CARTESIAN_POINT('Ctrl Pts',(0.704300982660464,-2.45411842762872,
0.0787150024977833));
#34597=CARTESIAN_POINT('Ctrl Pts',(0.700274469108872,-2.45079204224263,
0.15587784967814));
#34598=CARTESIAN_POINT('Ctrl Pts',(0.696247955557281,-2.44348687984151,
0.232658460786329));
#34599=CARTESIAN_POINT('Ctrl Pts',(0.653841677162244,-2.36655065535509,
1.04129350653413));
#34600=CARTESIAN_POINT('Ctrl Pts',(0.611435398767205,-1.84829648252061,
1.80753169553));
#34601=CARTESIAN_POINT('Ctrl Pts',(0.569029120372168,-1.12642923923531,
2.18058609450059));
#34602=CARTESIAN_POINT('Ctrl Pts',(0.529519413581445,-0.453869321141522,
2.52815891810498));
#34603=CARTESIAN_POINT('Ctrl Pts',(0.490009706790722,0.395437961240758,
2.53442654743051));
#34604=CARTESIAN_POINT('Ctrl Pts',(0.4505,1.07766119456972,2.20539011734829));
#34605=CARTESIAN_POINT('',(0.4505,-1.07508846035129,2.20207516956608));
#34606=CARTESIAN_POINT('Origin',(0.4505,0.,0.));
#34607=CARTESIAN_POINT('Ctrl Pts',(0.4505,-1.07508846035129,2.20207516956608));
#34608=CARTESIAN_POINT('Ctrl Pts',(0.492906278395038,-1.80850750214552,
1.84400821557093));
#34609=CARTESIAN_POINT('Ctrl Pts',(0.535312556790075,-2.34254929575026,
1.09374797713159));
#34610=CARTESIAN_POINT('Ctrl Pts',(0.577718835185113,-2.43734918119715,
0.288262827797322));
#34611=CARTESIAN_POINT('Ctrl Pts',(0.582703391386057,-2.44849223299838,
0.193583781490062));
#34612=CARTESIAN_POINT('Ctrl Pts',(0.587687947587001,-2.45356657398087,
0.0981417296316767));
#34613=CARTESIAN_POINT('Ctrl Pts',(0.592672503787945,-2.45282685237657,
0.00258448634202159));
#34614=CARTESIAN_POINT('Origin',(2.1,0.,0.));
#34615=CARTESIAN_POINT('',(1.50832749621205,-2.4473413370506,0.0014603139898775));
#34616=CARTESIAN_POINT('',(1.39267250378795,-2.44703157660636,0.00122755980643863));
#34617=CARTESIAN_POINT('',(2.1,-2.4505,-3.00099698131059E-16));
#34618=CARTESIAN_POINT('Ctrl Pts',(1.50832749621205,-2.4473413370506,0.0014603139898775));
#34619=CARTESIAN_POINT('Ctrl Pts',(1.49207198636402,-2.44903711369849,0.315247098410422));
#34620=CARTESIAN_POINT('Ctrl Pts',(1.47581647651599,-2.3930852952942,0.628451488488446));
#34621=CARTESIAN_POINT('Ctrl Pts',(1.45956096666796,-2.27670283532662,0.917306581367306));
#34622=CARTESIAN_POINT('Ctrl Pts',(1.41715468827292,-1.97309211847898,1.67085227750118));
#34623=CARTESIAN_POINT('Ctrl Pts',(1.37474840987789,-1.25822153135608,2.25868917842173));
#34624=CARTESIAN_POINT('Ctrl Pts',(1.33234213148285,-0.460215326170196,
2.41101669101588));
#34625=CARTESIAN_POINT('Ctrl Pts',(1.28993585308781,0.337790879015677,2.56334420361003));
#34626=CARTESIAN_POINT('Ctrl Pts',(1.24752957469277,1.21893270226453,2.28016232787779));
#34627=CARTESIAN_POINT('Ctrl Pts',(1.20512329629773,1.77875643166747,1.69141715907579));
#34628=CARTESIAN_POINT('Ctrl Pts',(1.1627170179027,2.33858016107041,1.10267199027379));
#34629=CARTESIAN_POINT('Ctrl Pts',(1.12031073950766,2.57708579662744,0.208363528402023));
#34630=CARTESIAN_POINT('Ctrl Pts',(1.07790446111262,2.384811555813,-0.580950218879841));
#34631=CARTESIAN_POINT('Ctrl Pts',(1.03549818271758,2.19253731499856,-1.3702639661617));
#34632=CARTESIAN_POINT('Ctrl Pts',(0.993091904322546,1.56948319781265,-2.05458299885366));
#34633=CARTESIAN_POINT('Ctrl Pts',(0.950685625927508,0.801608016347805,
-2.3199322416022));
#34634=CARTESIAN_POINT('Ctrl Pts',(0.90827934753247,0.0337328348829553,
-2.58528148435073));
#34635=CARTESIAN_POINT('Ctrl Pts',(0.865873069137432,-0.878963410860835,
-2.43166093715584));
#34636=CARTESIAN_POINT('Ctrl Pts',(0.823466790742394,-1.51750239566356,
-1.92933471230852));
#34637=CARTESIAN_POINT('Ctrl Pts',(0.785087025898947,-2.0954115404323,-1.47470480574751));
#34638=CARTESIAN_POINT('Ctrl Pts',(0.746707261055501,-2.44875466051846,
-0.734445229755698));
#34639=CARTESIAN_POINT('Ctrl Pts',(0.708327496212055,-2.45360913320878,
0.00150472093799672));
#34640=CARTESIAN_POINT('Ctrl Pts',(0.592672503787945,-2.45282685237657,
0.00258448634202159));
#34641=CARTESIAN_POINT('Ctrl Pts',(0.630094225982039,-2.44727336772092,
-0.714814709867619));
#34642=CARTESIAN_POINT('Ctrl Pts',(0.667515948176133,-2.11402153716249,
-1.43870644738133));
#34643=CARTESIAN_POINT('Ctrl Pts',(0.704937670370227,-1.56082513352308,
-1.89496977522306));
#34644=CARTESIAN_POINT('Ctrl Pts',(0.747343948765265,-0.933943223113065,
-2.41200716867997));
#34645=CARTESIAN_POINT('Ctrl Pts',(0.789750227160302,-0.0246214250039735,
-2.58537189536459));
#34646=CARTESIAN_POINT('Ctrl Pts',(0.83215650555534,0.749125781327214,-2.33722376134394));
#34647=CARTESIAN_POINT('Ctrl Pts',(0.874562783950378,1.5228729876584,-2.08907562732328));
#34648=CARTESIAN_POINT('Ctrl Pts',(0.916969062345416,2.16104560221169,-1.41941463259735));
#34649=CARTESIAN_POINT('Ctrl Pts',(0.959375340740454,2.37104638647788,-0.634742664260803));
#34650=CARTESIAN_POINT('Ctrl Pts',(1.00178161913549,2.58104717074407,0.149929304075739));
#34651=CARTESIAN_POINT('Ctrl Pts',(1.04418789753053,2.36287612472317,1.04961224602289));
#34652=CARTESIAN_POINT('Ctrl Pts',(1.08659417592557,1.81650481602726,1.6508958941018));
#34653=CARTESIAN_POINT('Ctrl Pts',(1.1290004543206,1.27013350733135,2.25217954218071));
#34654=CARTESIAN_POINT('Ctrl Pts',(1.17140673271564,0.395561935960428,2.55506389639137));
#34655=CARTESIAN_POINT('Ctrl Pts',(1.21381301111068,-0.405690332469361,
2.42076003474965));
#34656=CARTESIAN_POINT('Ctrl Pts',(1.25621928950572,-1.20694260089915,2.28645617310792));
#34657=CARTESIAN_POINT('Ctrl Pts',(1.29862556790075,-1.9348755663878,1.7149640956138));
#34658=CARTESIAN_POINT('Ctrl Pts',(1.34103184629579,-2.25541184946638,0.968477408375057));
#34659=CARTESIAN_POINT('Ctrl Pts',(1.35824539879318,-2.38552390704169,0.665463603209682));
#34660=CARTESIAN_POINT('Ctrl Pts',(1.37545895129056,-2.44850881837782,0.333615766579194));
#34661=CARTESIAN_POINT('Ctrl Pts',(1.39267250378795,-2.44703157660636,0.00122755980643863));
#34662=CARTESIAN_POINT('Origin',(2.1,0.,0.));
#34663=CARTESIAN_POINT('',(2.30832749621206,-2.44830822615452,-0.00194217634527288));
#34664=CARTESIAN_POINT('',(2.19267250378795,-2.44878095179287,-0.00208303942229182));
#34665=CARTESIAN_POINT('',(2.1,-2.4505,-3.00099698131059E-16));
#34666=CARTESIAN_POINT('Ctrl Pts',(2.30832749621206,-2.44830822615452,-0.00194217634527288));
#34667=CARTESIAN_POINT('Ctrl Pts',(2.27984299006758,-2.44424577234732,0.547360393912042));
#34668=CARTESIAN_POINT('Ctrl Pts',(2.25135848392311,-2.26154082184235,1.09911172701984));
#34669=CARTESIAN_POINT('Ctrl Pts',(2.22287397777864,-1.92217546127181,1.52645421544262));
#34670=CARTESIAN_POINT('Ctrl Pts',(2.1804676993836,-1.41694563966299,2.16265989308967));
#34671=CARTESIAN_POINT('Ctrl Pts',(2.13806142098857,-0.564497850275433,
2.52312911500327));
#34672=CARTESIAN_POINT('Ctrl Pts',(2.09565514259353,0.243894172460438,2.44240461641206));
#34673=CARTESIAN_POINT('Ctrl Pts',(2.05324886419849,1.05228619519631,2.36168011782086));
#34674=CARTESIAN_POINT('Ctrl Pts',(2.01084258580345,1.8166224512805,1.83976189872484));
#34675=CARTESIAN_POINT('Ctrl Pts',(1.96843630740841,2.18606878658389,1.11621194303221));
#34676=CARTESIAN_POINT('Ctrl Pts',(1.92603002901338,2.55551512188727,0.392661987339586));
#34677=CARTESIAN_POINT('Ctrl Pts',(1.88362375061834,2.53007153640987,-0.532519704949663));
#34678=CARTESIAN_POINT('Ctrl Pts',(1.8412174722233,2.12141763927363,-1.23467075668366));
#34679=CARTESIAN_POINT('Ctrl Pts',(1.79881119382826,1.7127637421374,-1.93682180841766));
#34680=CARTESIAN_POINT('Ctrl Pts',(1.75640491543323,0.920899533342334,-2.41594221959641));
#34681=CARTESIAN_POINT('Ctrl Pts',(1.71399863703819,0.109292333967081,-2.45211666963342));
#34682=CARTESIAN_POINT('Ctrl Pts',(1.67159235864315,-0.702314865408171,
-2.48829111967042));
#34683=CARTESIAN_POINT('Ctrl Pts',(1.62918608024811,-1.53366505536361,-2.08151960856568));
#34684=CARTESIAN_POINT('Ctrl Pts',(1.58677980185307,-2.00316472705514,-1.41850660733972));
#34685=CARTESIAN_POINT('Ctrl Pts',(1.56062903330607,-2.29269207328737,-1.00964499073661));
#34686=CARTESIAN_POINT('Ctrl Pts',(1.53447826475906,-2.44461328588265,-0.503338714106133));
#34687=CARTESIAN_POINT('Ctrl Pts',(1.50832749621205,-2.4473413370506,0.0014603139898775));
#34688=CARTESIAN_POINT('Ctrl Pts',(1.39267250378795,-2.44703157660636,0.00122755980643863));
#34689=CARTESIAN_POINT('Ctrl Pts',(1.4178652296856,-2.44486957390303,-0.48523593958517));
#34690=CARTESIAN_POINT('Ctrl Pts',(1.44305795558325,-2.30463286953165,-0.972856884742813));
#34691=CARTESIAN_POINT('Ctrl Pts',(1.46825068148091,-2.03467576323812,-1.37293946448399));
#34692=CARTESIAN_POINT('Ctrl Pts',(1.51065695987595,-1.58026379326277,-2.04638835312089));
#34693=CARTESIAN_POINT('Ctrl Pts',(1.55306323827098,-0.758300252643548,
-2.47180483341132));
#34694=CARTESIAN_POINT('Ctrl Pts',(1.59546951666602,0.0539184165626573,
-2.45395487916923));
#34695=CARTESIAN_POINT('Ctrl Pts',(1.63787579506106,0.866137085768862,-2.43610492492714));
#34696=CARTESIAN_POINT('Ctrl Pts',(1.6802820734561,1.66861088356205,-1.97498853615253));
#34697=CARTESIAN_POINT('Ctrl Pts',(1.72268835185113,2.09300840145503,-1.28224214439752));
#34698=CARTESIAN_POINT('Ctrl Pts',(1.76509463024617,2.51740591934801,-0.589495752642504));
#34699=CARTESIAN_POINT('Ctrl Pts',(1.80750090864121,2.56372715734077,0.334880642092917));
#34700=CARTESIAN_POINT('Ctrl Pts',(1.84990718703624,2.21070701757217,1.06658629749541));
#34701=CARTESIAN_POINT('Ctrl Pts',(1.89231346543128,1.85768687780357,1.79829195289791));
#34702=CARTESIAN_POINT('Ctrl Pts',(1.93471974382632,1.1053253602736,2.33732686896749));
#34703=CARTESIAN_POINT('Ctrl Pts',(1.97712602222136,0.298960721540154,2.43627696427715));
#34704=CARTESIAN_POINT('Ctrl Pts',(2.0195323006164,-0.507403917193297,2.53522705958681));
#34705=CARTESIAN_POINT('Ctrl Pts',(2.06193857901143,-1.36777167713024,2.19409233413654));
#34706=CARTESIAN_POINT('Ctrl Pts',(2.10434485740647,-1.88723228249209,1.56945243436612));
#34707=CARTESIAN_POINT('Ctrl Pts',(2.1337874062003,-2.24789218472075,1.13576687119931));
#34708=CARTESIAN_POINT('Ctrl Pts',(2.16322995499412,-2.44421839872437,0.565418142411997));
#34709=CARTESIAN_POINT('Ctrl Pts',(2.19267250378795,-2.44878095179287,-0.00208303942229182));
#34710=CARTESIAN_POINT('Origin',(2.1,0.,0.));
#34711=CARTESIAN_POINT('',(3.10832749621205,-2.45444621147543,-0.000567327939743623));
#34712=CARTESIAN_POINT('',(2.99267250378795,-2.45452615968528,-0.000257956296186217));
#34713=CARTESIAN_POINT('',(2.1,-2.4505,-3.00099698131059E-16));
#34714=CARTESIAN_POINT('Ctrl Pts',(3.10832749621205,-2.45444621147543,-0.000567327939743623));
#34715=CARTESIAN_POINT('Ctrl Pts',(3.06761399377114,-2.45192087847678,0.779588102337758));
#34716=CARTESIAN_POINT('Ctrl Pts',(3.02690049133023,-2.04779555002706,1.5619550530578));
#34717=CARTESIAN_POINT('Ctrl Pts',(2.98618698888932,-1.40912833240446,2.00973091739006));
#34718=CARTESIAN_POINT('Ctrl Pts',(2.94378071049429,-0.74390676686621,2.47612429607348));
#34719=CARTESIAN_POINT('Ctrl Pts',(2.90137443209925,0.175765592190175,2.57952508637236));
#34720=CARTESIAN_POINT('Ctrl Pts',(2.85896815370421,0.927875800169445,2.27241629395137));
#34721=CARTESIAN_POINT('Ctrl Pts',(2.81656187530917,1.67998600814872,1.96530750153038));
#34722=CARTESIAN_POINT('Ctrl Pts',(2.77415559691413,2.26453406505087,1.24768912638951));
#34723=CARTESIAN_POINT('Ctrl Pts',(2.73174931851909,2.41314815295225,0.448979332617362));
#34724=CARTESIAN_POINT('Ctrl Pts',(2.68934304012406,2.56176224085363,-0.349730461154791));
#34725=CARTESIAN_POINT('Ctrl Pts',(2.64693676172902,2.27444235975423,-1.22953167355824));
#34726=CARTESIAN_POINT('Ctrl Pts',(2.60453048333398,1.68310182647636,-1.78660792355543));
#34727=CARTESIAN_POINT('Ctrl Pts',(2.56212420493894,1.0917612931985,-2.34368417355261));
#34728=CARTESIAN_POINT('Ctrl Pts',(2.51971792654391,0.196400107742168,-2.57803546114354));
#34729=CARTESIAN_POINT('Ctrl Pts',(2.47731164814887,-0.592025137123773,
-2.3820859349775));
#34730=CARTESIAN_POINT('Ctrl Pts',(2.43490536975383,-1.38045038198972,-2.18613640881146));
#34731=CARTESIAN_POINT('Ctrl Pts',(2.39249909135879,-2.06193968626528,-1.55988606888843));
#34732=CARTESIAN_POINT('Ctrl Pts',(2.35009281296376,-2.323678411488,-0.790789832236671));
#34733=CARTESIAN_POINT('Ctrl Pts',(2.33617104071319,-2.40960594532532,-0.538299327276763));
#34734=CARTESIAN_POINT('Ctrl Pts',(2.32224926846262,-2.45029374615601,-0.270413226571201));
#34735=CARTESIAN_POINT('Ctrl Pts',(2.30832749621206,-2.44830822615452,-0.00194217634527288));
#34736=CARTESIAN_POINT('Ctrl Pts',(2.19267250378795,-2.44878095179287,-0.00208303942229182));
#34737=CARTESIAN_POINT('Ctrl Pts',(2.20563623338916,-2.45078987108465,-0.251957189965));
#34738=CARTESIAN_POINT('Ctrl Pts',(2.21859996299037,-2.41562169693219,-0.501279288473224));
#34739=CARTESIAN_POINT('Ctrl Pts',(2.23156369259159,-2.34093495686051,-0.738140446195743));
#34740=CARTESIAN_POINT('Ctrl Pts',(2.27396997098663,-2.09662357508032,-1.51294835289657));
#34741=CARTESIAN_POINT('Ctrl Pts',(2.31637624938166,-1.42944736073319,-2.15441909220764));
#34742=CARTESIAN_POINT('Ctrl Pts',(2.3587825277767,-0.645643695495165,-2.36811546388376));
#34743=CARTESIAN_POINT('Ctrl Pts',(2.40118880617174,0.138159969742868,-2.58181183555988));
#34744=CARTESIAN_POINT('Ctrl Pts',(2.44359508456678,1.0385910858718,-2.36773383960104));
#34745=CARTESIAN_POINT('Ctrl Pts',(2.48600136296181,1.64235124726471,-1.82414509847746));
#34746=CARTESIAN_POINT('Ctrl Pts',(2.52840764135685,2.24611140865762,-1.28055635735387));
#34747=CARTESIAN_POINT('Ctrl Pts',(2.57081391975189,2.55320061531452,-0.407456871065538));
#34748=CARTESIAN_POINT('Ctrl Pts',(2.61322019814693,2.42265969342523,0.394400630578321));
#34749=CARTESIAN_POINT('Ctrl Pts',(2.65562647654196,2.29211877153594,1.19625813222218));
#34750=CARTESIAN_POINT('Ctrl Pts',(2.698032754937,1.72394772110046,1.92687364922157));
#34751=CARTESIAN_POINT('Ctrl Pts',(2.74043903333204,0.978946913942611,2.25088694187707));
#34752=CARTESIAN_POINT('Ctrl Pts',(2.78284531172708,0.233946106784758,2.57490023453258));
#34753=CARTESIAN_POINT('Ctrl Pts',(2.82525159012211,-0.687884457095468,
2.4923113028442));
#34754=CARTESIAN_POINT('Ctrl Pts',(2.86765786851715,-1.36343705087406,2.04103923356386));
#34755=CARTESIAN_POINT('Ctrl Pts',(2.90932941360742,-2.02728498655577,1.59758592677255));
#34756=CARTESIAN_POINT('Ctrl Pts',(2.95100095869768,-2.45331507036201,0.798114451695043));
#34757=CARTESIAN_POINT('Ctrl Pts',(2.99267250378795,-2.45452615968528,-0.000257956296186217));
#34758=CARTESIAN_POINT('Origin',(-1.02854511860477,0.,0.));
#34759=CARTESIAN_POINT('',(3.37145488139523,-1.99796228538691,-0.000461814898120527));
#34760=CARTESIAN_POINT('',(3.52954511860477,-1.99388364589384,0.00171352076686206));
#34761=CARTESIAN_POINT('',(-1.02854511860477,-1.99475,-1.3903373121373E-14));
#34762=CARTESIAN_POINT('',(3.7495,1.96855338775712,-0.342146149675743));
#34763=CARTESIAN_POINT('Ctrl Pts',(3.37145488139523,-1.9979622853869,-0.00046181489812086));
#34764=CARTESIAN_POINT('Ctrl Pts',(3.37314765734935,-1.99804775533437,-0.0268661915402383));
#34765=CARTESIAN_POINT('Ctrl Pts',(3.41724671169852,-1.98555193750958,-0.714654081742635));
#34766=CARTESIAN_POINT('Ctrl Pts',(3.50375204444272,-1.19567276206334,-2.03345149280708));
#34767=CARTESIAN_POINT('Ctrl Pts',(3.62807430802352,1.01077702469923,-2.10391583542276));
#34768=CARTESIAN_POINT('Ctrl Pts',(3.70999029320928,1.8598858594405,-0.9490459619713));
#34769=CARTESIAN_POINT('Ctrl Pts',(3.7495,1.96858208699144,-0.342145191103274));
#34770=CARTESIAN_POINT('',(3.7495,0.311349471200418,-1.97030177112117));
#34771=CARTESIAN_POINT('Origin',(3.7495,0.,0.));
#34772=CARTESIAN_POINT('Ctrl Pts',(3.52954511860477,-1.99388364589384,0.00171352076686202));
#34773=CARTESIAN_POINT('Ctrl Pts',(3.56045713400815,-1.98914408542672,-0.483238452536014));
#34774=CARTESIAN_POINT('Ctrl Pts',(3.63377542780655,-1.56621865433236,-1.64019501966093));
#34775=CARTESIAN_POINT('Ctrl Pts',(3.70709372160496,-0.344875555534673,
-2.07399924429869));
#34776=CARTESIAN_POINT('Ctrl Pts',(3.7495,0.311349471200418,-1.97030177112117));
#34777=CARTESIAN_POINT('Origin',(-1.02854511860477,0.,0.));
#34778=CARTESIAN_POINT('',(2.57145488139523,-1.99296585762976,-0.00158096562527621));
#34779=CARTESIAN_POINT('',(2.72954511860477,-1.99802736463261,-0.000209980951578204));
#34780=CARTESIAN_POINT('',(-1.02854511860477,-1.99475,-1.3903373121373E-14));
#34781=CARTESIAN_POINT('Ctrl Pts',(2.57145488139523,-1.99296585762976,-0.00158096562527653));
#34782=CARTESIAN_POINT('Ctrl Pts',(2.58537665364579,-1.99458210575176,-0.22012111148864));
#34783=CARTESIAN_POINT('Ctrl Pts',(2.6417047042914,-1.86057489097072,-1.10241677508306));
#34784=CARTESIAN_POINT('Ctrl Pts',(2.74043903333204,-0.568966582236417,
-2.28933216365562));
#34785=CARTESIAN_POINT('Ctrl Pts',(2.86765786851715,1.61755256653611,-1.71703398256359));
#34786=CARTESIAN_POINT('Ctrl Pts',(2.99487670370227,2.31920284136536,0.43148689290074));
#34787=CARTESIAN_POINT('Ctrl Pts',(3.12209553888738,0.891705714445654,2.18394874208935));
#34788=CARTESIAN_POINT('Ctrl Pts',(3.24762159811837,-1.32429877248386,1.93479847352036));
#34789=CARTESIAN_POINT('Ctrl Pts',(3.33074137895432,-1.99590662001288,0.634598395077826));
#34790=CARTESIAN_POINT('Ctrl Pts',(3.37145488139523,-1.9979622853869,-0.00046181489812086));
#34791=CARTESIAN_POINT('Ctrl Pts',(2.72954511860477,-1.99802736463261,-0.000209980951578455));
#34792=CARTESIAN_POINT('Ctrl Pts',(2.73027985190955,-1.99804474664541,-0.0116685242216074));
#34793=CARTESIAN_POINT('Ctrl Pts',(2.77342086360936,-1.99275319078551,-0.684458429783003));
#34794=CARTESIAN_POINT('Ctrl Pts',(2.85896815370421,-1.24161073233134,-2.00578545294822));
#34795=CARTESIAN_POINT('Ctrl Pts',(2.98618698888932,1.01505102673121,-2.12930526437765));
#34796=CARTESIAN_POINT('Ctrl Pts',(3.11340582407443,2.34023742749476,-0.298347997134086));
#34797=CARTESIAN_POINT('Ctrl Pts',(3.24062465925955,1.51640407537933,1.80695219210931));
#34798=CARTESIAN_POINT('Ctrl Pts',(3.36784349444466,-0.698217180620254,
2.25257951257453));
#34799=CARTESIAN_POINT('Ctrl Pts',(3.4641503142264,-1.8913724236262,1.02579681025012));
#34800=CARTESIAN_POINT('Ctrl Pts',(3.51805085561311,-1.99564599473338,0.182037108431196));
#34801=CARTESIAN_POINT('Ctrl Pts',(3.52954511860477,-1.99388364589384,0.00171352076686202));
#34802=CARTESIAN_POINT('Origin',(-1.02854511860477,0.,0.));
#34803=CARTESIAN_POINT('',(1.77145488139523,-1.99217879293274,0.0011887212125215));
#34804=CARTESIAN_POINT('',(1.92954511860477,-1.9933506645945,-0.0016956306417637));
#34805=CARTESIAN_POINT('',(-1.02854511860477,-1.99475,-1.3903373121373E-14));
#34806=CARTESIAN_POINT('Ctrl Pts',(1.77145488139523,-1.99217879293274,0.00118872121252139));
#34807=CARTESIAN_POINT('Ctrl Pts',(1.79760564994223,-1.98995811141171,-0.409726545587932));
#34808=CARTESIAN_POINT('Ctrl Pts',(1.86616269688428,-1.66575302028294,-1.49020154805744));
#34809=CARTESIAN_POINT('Ctrl Pts',(1.97712602222136,0.105037018421004,-2.35663178238676));
#34810=CARTESIAN_POINT('Ctrl Pts',(2.10434485740647,2.03881110186596,-1.18659451627925));
#34811=CARTESIAN_POINT('Ctrl Pts',(2.23156369259159,2.1009456770111,1.07274787999985));
#34812=CARTESIAN_POINT('Ctrl Pts',(2.3587825277767,0.234396303221342,2.34729964601711));
#34813=CARTESIAN_POINT('Ctrl Pts',(2.47207959071125,-1.61951967361292,1.56334588605397));
#34814=CARTESIAN_POINT('Ctrl Pts',(2.54297037525076,-1.98965894894504,0.445560965417686));
#34815=CARTESIAN_POINT('Ctrl Pts',(2.57145488139523,-1.99296585762976,-0.00158096562527653));
#34816=CARTESIAN_POINT('Ctrl Pts',(1.92954511860477,-1.9933506645945,-0.00169563064176386));
#34817=CARTESIAN_POINT('Ctrl Pts',(1.94250884820599,-1.9949859601494,-0.205097573835013));
#34818=CARTESIAN_POINT('Ctrl Pts',(1.99787885620224,-1.87271362382115,-1.0719380117463));
#34819=CARTESIAN_POINT('Ctrl Pts',(2.09565514259353,-0.620502089064916,
-2.27590338356333));
#34820=CARTESIAN_POINT('Ctrl Pts',(2.22287397777864,1.57839809730298,-1.75311364786995));
#34821=CARTESIAN_POINT('Ctrl Pts',(2.35009281296375,2.32832610584676,0.379041259626889));
#34822=CARTESIAN_POINT('Ctrl Pts',(2.47731164814887,0.940822490842265,2.16324281343369));
#34823=CARTESIAN_POINT('Ctrl Pts',(2.60379575002921,-1.29733504359323,1.96272110482245));
#34824=CARTESIAN_POINT('Ctrl Pts',(2.68787357351451,-1.99704151667196,0.649679168544651));
#34825=CARTESIAN_POINT('Ctrl Pts',(2.72954511860477,-1.99802736463261,-0.000209980951578455));
#34826=CARTESIAN_POINT('Origin',(-1.02854511860477,0.,0.));
#34827=CARTESIAN_POINT('',(0.971454881395227,-1.99728088898928,0.00122486924751956));
#34828=CARTESIAN_POINT('',(1.12954511860477,-1.99192664249562,0.000999255222959294));
#34829=CARTESIAN_POINT('',(-1.02854511860477,-1.99475,-1.3903373121373E-14));
#34830=CARTESIAN_POINT('Ctrl Pts',(0.971454881395227,-1.99728088898927,
0.00122486924751962));
#34831=CARTESIAN_POINT('Ctrl Pts',(1.00983464623867,-1.99332926303579,-0.597851304654232));
#34832=CARTESIAN_POINT('Ctrl Pts',(1.09062068947716,-1.38789856934239,-1.86623844205377));
#34833=CARTESIAN_POINT('Ctrl Pts',(1.21381301111068,0.770409879037013,-2.22951431439528));
#34834=CARTESIAN_POINT('Ctrl Pts',(1.34103184629579,2.2919408322179,-0.558371212421443));
#34835=CARTESIAN_POINT('Ctrl Pts',(1.4682506814809,1.70949751469815,1.62557712993974));
#34836=CARTESIAN_POINT('Ctrl Pts',(1.59546951666602,-0.442297203023523,
2.3171221778282));
#34837=CARTESIAN_POINT('Ctrl Pts',(1.69653758330413,-1.82919670899801,1.17667700891804));
#34838=CARTESIAN_POINT('Ctrl Pts',(1.7551993715472,-1.99355918488066,0.256616669885401));
#34839=CARTESIAN_POINT('Ctrl Pts',(1.77145488139523,-1.99217879293274,0.00118872121252139));
#34840=CARTESIAN_POINT('Ctrl Pts',(1.12954511860477,-1.99192664249562,0.000999255222959156));
#34841=CARTESIAN_POINT('Ctrl Pts',(1.15473784450243,-1.99016673435751,-0.394990569470533));
#34842=CARTESIAN_POINT('Ctrl Pts',(1.22233684879512,-1.68385713906353,-1.46006818262196));
#34843=CARTESIAN_POINT('Ctrl Pts',(1.33234213148285,0.0518230335398809,
-2.35838898816837));
#34844=CARTESIAN_POINT('Ctrl Pts',(1.45956096666796,2.01150629183162,-1.23231849254524));
#34845=CARTESIAN_POINT('Ctrl Pts',(1.58677980185307,2.12462519346728,1.02505732471468));
#34846=CARTESIAN_POINT('Ctrl Pts',(1.71399863703819,0.287318761604926,2.341408965804));
#34847=CARTESIAN_POINT('Ctrl Pts',(1.82825374262209,-1.59964409149406,1.59323058813681));
#34848=CARTESIAN_POINT('Ctrl Pts',(1.90010256981095,-1.98963666633563,0.46026028956389));
#34849=CARTESIAN_POINT('Ctrl Pts',(1.92954511860477,-1.9933506645945,-0.00169563064176386));
#34850=CARTESIAN_POINT('Origin',(3.7495,5.69858952725515E-16,8.58067791224701E-17));
#34851=CARTESIAN_POINT('',(3.7495,-0.778675485261968,2.32349192782158));
#34852=CARTESIAN_POINT('Ctrl Pts',(3.7495,1.96858208699144,-0.342145191103275));
#34853=CARTESIAN_POINT('Ctrl Pts',(3.7495,1.9815616872834,-0.298310884910423));
#34854=CARTESIAN_POINT('Ctrl Pts',(3.7495,1.99290809419775,-0.254078248249005));
#34855=CARTESIAN_POINT('Ctrl Pts',(3.7495,2.00257142811677,-0.209519371139262));
#34856=CARTESIAN_POINT('Ctrl Pts',(3.7495,2.01774911827413,-0.139533087295686));
#34857=CARTESIAN_POINT('Ctrl Pts',(3.7495,2.02877766589333,-0.0687429867827845));
#34858=CARTESIAN_POINT('Ctrl Pts',(3.7495,2.0358403959562,0.00254783820095801));
#34859=CARTESIAN_POINT('Ctrl Pts',(3.7495,2.03975568900501,0.0420685998636354));
#34860=CARTESIAN_POINT('Ctrl Pts',(3.7495,2.04245137734559,0.0817436825706553));
#34861=CARTESIAN_POINT('Ctrl Pts',(3.7495,2.04395245361958,0.121523911179525));
#34862=CARTESIAN_POINT('Ctrl Pts',(3.7495,2.04469239255816,0.14113313467024));
#34863=CARTESIAN_POINT('Ctrl Pts',(3.7495,2.04514198673599,0.1607679282988));
#34864=CARTESIAN_POINT('Ctrl Pts',(3.7495,2.04530383971613,0.180422499284288));
#34865=CARTESIAN_POINT('Ctrl Pts',(3.7495,2.04542150599878,0.194711271125375));
#34866=CARTESIAN_POINT('Ctrl Pts',(3.7495,2.04538700750185,0.209000770084867));
#34867=CARTESIAN_POINT('Ctrl Pts',(3.7495,2.04520188976334,0.223288377519502));
#34868=CARTESIAN_POINT('Ctrl Pts',(3.7495,2.04422777843955,0.298471449137185));
#34869=CARTESIAN_POINT('Ctrl Pts',(3.7495,2.03908721806814,0.373602904565653));
#34870=CARTESIAN_POINT('Ctrl Pts',(3.7495,2.02997465441022,0.448351081788569));
#34871=CARTESIAN_POINT('Ctrl Pts',(3.7495,2.02256734831719,0.509111439616568));
#34872=CARTESIAN_POINT('Ctrl Pts',(3.7495,2.01253450727956,0.569619224635133));
#34873=CARTESIAN_POINT('Ctrl Pts',(3.7495,1.99995593276109,0.629702334442525));
#34874=CARTESIAN_POINT('Ctrl Pts',(3.7495,1.99497851113414,0.653477601642343));
#34875=CARTESIAN_POINT('Ctrl Pts',(3.7495,1.98960223154056,0.677186401041374));
#34876=CARTESIAN_POINT('Ctrl Pts',(3.7495,1.98383111448107,0.700818115169424));
#34877=CARTESIAN_POINT('Ctrl Pts',(3.7495,1.9797346628459,0.717592367534078));
#34878=CARTESIAN_POINT('Ctrl Pts',(3.7495,1.97543835661824,0.73433067219556));
#34879=CARTESIAN_POINT('Ctrl Pts',(3.7495,1.97095036387965,0.75100507213264));
#34880=CARTESIAN_POINT('Ctrl Pts',(3.7495,1.95073133439056,0.826125555537453));
#34881=CARTESIAN_POINT('Ctrl Pts',(3.7495,1.92660313283638,0.900047712653736));
#34882=CARTESIAN_POINT('Ctrl Pts',(3.7495,1.89876242591588,0.972434182739083));
#34883=CARTESIAN_POINT('Ctrl Pts',(3.7495,1.87039439526001,1.0461917065087));
#34884=CARTESIAN_POINT('Ctrl Pts',(3.7495,1.83817184686105,1.11835584035847));
#34885=CARTESIAN_POINT('Ctrl Pts',(3.7495,1.80224930993342,1.18857395679423));
#34886=CARTESIAN_POINT('Ctrl Pts',(3.7495,1.7760002690807,1.23988320064403));
#34887=CARTESIAN_POINT('Ctrl Pts',(3.7495,1.74777452061065,1.29015354758491));
#34888=CARTESIAN_POINT('Ctrl Pts',(3.7495,1.71761511908426,1.33924389352241));
#34889=CARTESIAN_POINT('Ctrl Pts',(3.7495,1.69499556793946,1.37606165297554));
#34890=CARTESIAN_POINT('Ctrl Pts',(3.7495,1.67128803582605,1.41221561571887));
#34891=CARTESIAN_POINT('Ctrl Pts',(3.7495,1.64650557338506,1.44764383520813));
#34892=CARTESIAN_POINT('Ctrl Pts',(3.7495,1.63899129825552,1.4583860037568));
#34893=CARTESIAN_POINT('Ctrl Pts',(3.7495,1.63137694759429,1.46906310763164));
#34894=CARTESIAN_POINT('Ctrl Pts',(3.7495,1.62366670212987,1.47966802512963));
#34895=CARTESIAN_POINT('Ctrl Pts',(3.7495,1.57597942677249,1.54525862444354));
#34896=CARTESIAN_POINT('Ctrl Pts',(3.7495,1.5247886717997,1.60787005386699));
#34897=CARTESIAN_POINT('Ctrl Pts',(3.7495,1.47026968124208,1.66714346245527));
#34898=CARTESIAN_POINT('Ctrl Pts',(3.7495,1.44638830509851,1.69310745319189));
#34899=CARTESIAN_POINT('Ctrl Pts',(3.7495,1.42186764705416,1.71843085924667));
#34900=CARTESIAN_POINT('Ctrl Pts',(3.7495,1.39671939232244,1.74308270436089));
#34901=CARTESIAN_POINT('Ctrl Pts',(3.7495,1.34130534744921,1.79740291329546));
#34902=CARTESIAN_POINT('Ctrl Pts',(3.7495,1.28284699014363,1.8484646870851));
#34903=CARTESIAN_POINT('Ctrl Pts',(3.7495,1.22168664345893,1.89625311771161));
#34904=CARTESIAN_POINT('Ctrl Pts',(3.7495,1.15924467146654,1.94504296290533));
#34905=CARTESIAN_POINT('Ctrl Pts',(3.7495,1.09398565883421,1.99042130918484));
#34906=CARTESIAN_POINT('Ctrl Pts',(3.7495,1.02623383171228,2.03233611927841));
#34907=CARTESIAN_POINT('Ctrl Pts',(3.7495,1.01504933682572,2.03925543052176));
#34908=CARTESIAN_POINT('Ctrl Pts',(3.7495,1.00379683470936,2.04608026748763));
#34909=CARTESIAN_POINT('Ctrl Pts',(3.7495,0.992477701009896,2.05281028972857));
#34910=CARTESIAN_POINT('Ctrl Pts',(3.7495,0.98172367113139,2.05920431794519));
#34911=CARTESIAN_POINT('Ctrl Pts',(3.7495,0.970918002482417,2.0655077016547));
#34912=CARTESIAN_POINT('Ctrl Pts',(3.7495,0.960062601834612,2.07172027426472));
#34913=CARTESIAN_POINT('Ctrl Pts',(3.7495,0.889742058929685,2.11196489470268));
#34914=CARTESIAN_POINT('Ctrl Pts',(3.7495,0.817332785201951,2.1484046376665));
#34915=CARTESIAN_POINT('Ctrl Pts',(3.7495,0.743220237068545,2.18103885646569));
#34916=CARTESIAN_POINT('Ctrl Pts',(3.7495,0.667662831350121,2.21430929409355));
#34917=CARTESIAN_POINT('Ctrl Pts',(3.7495,0.590334370784013,2.24362483808424));
#34918=CARTESIAN_POINT('Ctrl Pts',(3.7495,0.511603026210655,2.26894693390449));
#34919=CARTESIAN_POINT('Ctrl Pts',(3.7495,0.432317848910233,2.29444715706982));
#34920=CARTESIAN_POINT('Ctrl Pts',(3.7495,0.351609102256153,2.31589797265474));
#34921=CARTESIAN_POINT('Ctrl Pts',(3.7495,0.269824604998954,2.33321541018852));
#34922=CARTESIAN_POINT('Ctrl Pts',(3.7495,0.237358854089674,2.34008986234283));
#34923=CARTESIAN_POINT('Ctrl Pts',(3.7495,0.204723346095625,2.34631243924816));
#34924=CARTESIAN_POINT('Ctrl Pts',(3.7495,0.171939102120644,2.35187572830449));
#34925=CARTESIAN_POINT('Ctrl Pts',(3.7495,0.155509674618924,2.35466370335408));
#34926=CARTESIAN_POINT('Ctrl Pts',(3.7495,0.139039506256638,2.35728648113795));
#34927=CARTESIAN_POINT('Ctrl Pts',(3.7495,0.122556884830378,2.35973950905647));
#34928=CARTESIAN_POINT('Ctrl Pts',(3.7495,0.0376196930479621,2.3723802958206));
#34929=CARTESIAN_POINT('Ctrl Pts',(3.7495,-0.0477770629941537,2.38054113558466));
#34930=CARTESIAN_POINT('Ctrl Pts',(3.7495,-0.133242592282125,2.38419061215778));
#34931=CARTESIAN_POINT('Ctrl Pts',(3.7495,-0.21883889220705,2.38784567278777));
#34932=CARTESIAN_POINT('Ctrl Pts',(3.7495,-0.304505141737865,2.38697591690384));
#34933=CARTESIAN_POINT('Ctrl Pts',(3.7495,-0.389871608999167,2.38150287230091));
#34934=CARTESIAN_POINT('Ctrl Pts',(3.7495,-0.473426854966115,2.37614594934677));
#34935=CARTESIAN_POINT('Ctrl Pts',(3.7495,-0.55669585319343,2.36637916882364));
#34936=CARTESIAN_POINT('Ctrl Pts',(3.7495,-0.639339556196431,2.35208041838678));
#34937=CARTESIAN_POINT('Ctrl Pts',(3.7495,-0.686004718048208,2.34400656061943));
#34938=CARTESIAN_POINT('Ctrl Pts',(3.7495,-0.732470576108049,2.33448685588941));
#34939=CARTESIAN_POINT('Ctrl Pts',(3.7495,-0.778675485261984,2.32349192782157));
#34940=CARTESIAN_POINT('',(3.7495,-2.4505,-3.00099698131059E-16));
#34941=CARTESIAN_POINT('Origin',(3.7495,0.,0.));
#34942=CARTESIAN_POINT('',(3.7495,-2.31305386802746,0.815353369809073));
#34943=CARTESIAN_POINT('Origin',(3.7495,0.,0.));
#34944=CARTESIAN_POINT('Ctrl Pts',(3.7495,-2.31513335459631,0.81563149263664));
#34945=CARTESIAN_POINT('Ctrl Pts',(3.7495,-2.32908511219393,0.761794304485864));
#34946=CARTESIAN_POINT('Ctrl Pts',(3.7495,-2.34105243639297,0.707526344258663));
#34947=CARTESIAN_POINT('Ctrl Pts',(3.7495,-2.35095796922772,0.652895508310378));
#34948=CARTESIAN_POINT('Ctrl Pts',(3.7495,-2.36615894451881,0.569059332989447));
#34949=CARTESIAN_POINT('Ctrl Pts',(3.7495,-2.37650681260459,0.484368010711472));
#34950=CARTESIAN_POINT('Ctrl Pts',(3.7495,-2.38213543171266,0.399197491499006));
#34951=CARTESIAN_POINT('Ctrl Pts',(3.7495,-2.38498599869696,0.356063595699415));
#34952=CARTESIAN_POINT('Ctrl Pts',(3.7495,-2.38662532033442,0.312806868142191));
#34953=CARTESIAN_POINT('Ctrl Pts',(3.7495,-2.38706590699035,0.269477264460517));
#34954=CARTESIAN_POINT('Ctrl Pts',(3.7495,-2.38734080394354,0.242442455587761));
#34955=CARTESIAN_POINT('Ctrl Pts',(3.7495,-2.38714897815231,0.215379296141133));
#34956=CARTESIAN_POINT('Ctrl Pts',(3.7495,-2.38649286933422,0.18830018295618));
#34957=CARTESIAN_POINT('Ctrl Pts',(3.7495,-2.38607609390504,0.171098906722011));
#34958=CARTESIAN_POINT('Ctrl Pts',(3.7495,-2.3854721526339,0.153900233382592));
#34959=CARTESIAN_POINT('Ctrl Pts',(3.7495,-2.38468248454918,0.136712098302334));
#34960=CARTESIAN_POINT('Ctrl Pts',(3.7495,-2.38078339237081,0.0518433738995889));
#34961=CARTESIAN_POINT('Ctrl Pts',(3.7495,-2.37235943327698,-0.032807596098823));
#34962=CARTESIAN_POINT('Ctrl Pts',(3.7495,-2.35953861383588,-0.116866026728083));
#34963=CARTESIAN_POINT('Ctrl Pts',(3.7495,-2.34969292129715,-0.181418333003472));
#34964=CARTESIAN_POINT('Ctrl Pts',(3.7495,-2.337253079783,-0.245621176759048));
#34965=CARTESIAN_POINT('Ctrl Pts',(3.7495,-2.32225795639588,-0.309296437066621));
#34966=CARTESIAN_POINT('Ctrl Pts',(3.7495,-2.31481601340137,-0.340897888094137));
#34967=CARTESIAN_POINT('Ctrl Pts',(3.7495,-2.3067444494143,-0.372369249750108));
#34968=CARTESIAN_POINT('Ctrl Pts',(3.7495,-2.29804664763249,-0.403687743159158));
#34969=CARTESIAN_POINT('Ctrl Pts',(3.7495,-2.2928307316521,-0.422468882848428));
#34970=CARTESIAN_POINT('Ctrl Pts',(3.7495,-2.28738798603973,-0.441199905116059));
#34971=CARTESIAN_POINT('Ctrl Pts',(3.7495,-2.28172827744347,-0.459846435299733));
#34972=CARTESIAN_POINT('Ctrl Pts',(3.7495,-2.25757253969978,-0.539430160377721));
#34973=CARTESIAN_POINT('Ctrl Pts',(3.7495,-2.22944528228881,-0.617567924839354));
#34974=CARTESIAN_POINT('Ctrl Pts',(3.7495,-2.19746473876446,-0.693910868197669));
#34975=CARTESIAN_POINT('Ctrl Pts',(3.7495,-2.16615935321421,-0.76864209576586));
#34976=CARTESIAN_POINT('Ctrl Pts',(3.7495,-2.13116109945797,-0.84165425052456));
#34977=CARTESIAN_POINT('Ctrl Pts',(3.7495,-2.09254034740989,-0.912592837701785));
#34978=CARTESIAN_POINT('Ctrl Pts',(3.7495,-2.05476766251083,-0.981973695363329));
#34979=CARTESIAN_POINT('Ctrl Pts',(3.7495,-2.01352934821663,-1.04937167195347));
#34980=CARTESIAN_POINT('Ctrl Pts',(3.7495,-1.96885960929661,-1.11441869429856));
#34981=CARTESIAN_POINT('Ctrl Pts',(3.7495,-1.95318632744929,-1.13724175839501));
#34982=CARTESIAN_POINT('Ctrl Pts',(3.7495,-1.93709034646413,-1.1597750203898));
#34983=CARTESIAN_POINT('Ctrl Pts',(3.7495,-1.92057235305432,-1.18200127152593));
#34984=CARTESIAN_POINT('Ctrl Pts',(3.7495,-1.91106338439778,-1.19479633204945));
#34985=CARTESIAN_POINT('Ctrl Pts',(3.7495,-1.90141455374021,-1.20748963577181));
#34986=CARTESIAN_POINT('Ctrl Pts',(3.7495,-1.8916259361486,-1.22007778499248));
#34987=CARTESIAN_POINT('Ctrl Pts',(3.7495,-1.88396079263015,-1.22993514937567));
#34988=CARTESIAN_POINT('Ctrl Pts',(3.7495,-1.87621545865249,-1.23972090682631));
#34989=CARTESIAN_POINT('Ctrl Pts',(3.7495,-1.86839145414301,-1.24943232120233));
#34990=CARTESIAN_POINT('Ctrl Pts',(3.7495,-1.81941381572349,-1.31022499345529));
#34991=CARTESIAN_POINT('Ctrl Pts',(3.7495,-1.76734121286946,-1.36812667523011));
#34992=CARTESIAN_POINT('Ctrl Pts',(3.7495,-1.71224095284068,-1.42281218692403));
#34993=CARTESIAN_POINT('Ctrl Pts',(3.7495,-1.69359197104109,-1.44132079490062));
#34994=CARTESIAN_POINT('Ctrl Pts',(3.7495,-1.67459588005271,-1.45946065497124));
#34995=CARTESIAN_POINT('Ctrl Pts',(3.7495,-1.65525445681708,-1.4772180716962));
#34996=CARTESIAN_POINT('Ctrl Pts',(3.7495,-1.59693556290941,-1.53076081720367));
#34997=CARTESIAN_POINT('Ctrl Pts',(3.7495,-1.53547843782113,-1.58083011632459));
#34998=CARTESIAN_POINT('Ctrl Pts',(3.7495,-1.47124006561597,-1.62733004442714));
#34999=CARTESIAN_POINT('Ctrl Pts',(3.7495,-1.40824533562139,-1.67292974309684));
#35000=CARTESIAN_POINT('Ctrl Pts',(3.7495,-1.34257497746214,-1.71509694250743));
#35001=CARTESIAN_POINT('Ctrl Pts',(3.7495,-1.27455552459032,-1.75369441034441));
#35002=CARTESIAN_POINT('Ctrl Pts',(3.7495,-1.25783784098724,-1.76318081795188));
#35003=CARTESIAN_POINT('Ctrl Pts',(3.7495,-1.24097196291893,-1.77245454468573));
#35004=CARTESIAN_POINT('Ctrl Pts',(3.7495,-1.2239962012115,-1.78149579204408));
#35005=CARTESIAN_POINT('Ctrl Pts',(3.7495,-1.15532479262889,-1.818070008986));
#35006=CARTESIAN_POINT('Ctrl Pts',(3.7495,-1.0847804637132,-1.85089071870811));
#35007=CARTESIAN_POINT('Ctrl Pts',(3.7495,-1.01271311544069,-1.87989331065926));
#35008=CARTESIAN_POINT('Ctrl Pts',(3.7495,-0.940712023936066,-1.90886923841299));
#35009=CARTESIAN_POINT('Ctrl Pts',(3.7495,-0.867189652651409,-1.9340341824166));
#35010=CARTESIAN_POINT('Ctrl Pts',(3.7495,-0.792485063082482,-1.95527294001421));
#35011=CARTESIAN_POINT('Ctrl Pts',(3.7495,-0.719036476900967,-1.97615461176689));
#35012=CARTESIAN_POINT('Ctrl Pts',(3.7495,-0.644444141266421,-1.99324098626649));
#35013=CARTESIAN_POINT('Ctrl Pts',(3.7495,-0.56903562000595,-2.00637298650572));
#35014=CARTESIAN_POINT('Ctrl Pts',(3.7495,-0.540403830116529,-2.01135906321685));
#35015=CARTESIAN_POINT('Ctrl Pts',(3.7495,-0.511654504155911,-2.0157745477122));
#35016=CARTESIAN_POINT('Ctrl Pts',(3.7495,-0.482806204745629,-2.01960882217606));
#35017=CARTESIAN_POINT('Ctrl Pts',(3.7495,-0.470508509360357,-2.02124332890068));
#35018=CARTESIAN_POINT('Ctrl Pts',(3.7495,-0.458192645595391,-2.0227721434037));
#35019=CARTESIAN_POINT('Ctrl Pts',(3.7495,-0.445874680385831,-2.02419294658075));
#35020=CARTESIAN_POINT('Ctrl Pts',(3.7495,-0.371370875225623,-2.03278651226092));
#35021=CARTESIAN_POINT('Ctrl Pts',(3.7495,-0.29665767767233,-2.03745123135788));
#35022=CARTESIAN_POINT('Ctrl Pts',(3.7495,-0.222044113785007,-2.03809073316757));
#35023=CARTESIAN_POINT('Ctrl Pts',(3.7495,-0.148642426162284,-2.03871984816521));
#35024=CARTESIAN_POINT('Ctrl Pts',(3.7495,-0.0753363029714272,-2.03545337277455));
#35025=CARTESIAN_POINT('Ctrl Pts',(3.7495,-0.00243027506051708,-2.02815091108686));
#35026=CARTESIAN_POINT('Ctrl Pts',(3.7495,0.0681397525587181,-2.02108242940222));
#35027=CARTESIAN_POINT('Ctrl Pts',(3.7495,0.138335550220238,-2.01023226935319));
#35028=CARTESIAN_POINT('Ctrl Pts',(3.7495,0.207860443914689,-1.99542917781665));
#35029=CARTESIAN_POINT('Ctrl Pts',(3.7495,0.242537247572915,-1.98804586701285));
#35030=CARTESIAN_POINT('Ctrl Pts',(3.7495,0.277046768135923,-1.97967850842822));
#35031=CARTESIAN_POINT('Ctrl Pts',(3.7495,0.311349471200403,-1.97030177112117));
#35032=CARTESIAN_POINT('Ctrl Pts',(0.187372614816828,-0.875140871775444,
1.79252782880716));
#35033=CARTESIAN_POINT('Ctrl Pts',(0.229778893211866,-1.47215684142207,
1.50105504509697));
#35034=CARTESIAN_POINT('Ctrl Pts',(0.314591450001942,-2.34159562354249,
0.279605046625738));
#35035=CARTESIAN_POINT('Ctrl Pts',(0.441810285187055,-1.5004500718559,-1.82229423022658));
#35036=CARTESIAN_POINT('Ctrl Pts',(0.569029120372168,0.720161627933661,
-2.24566001911148));
#35037=CARTESIAN_POINT('Ctrl Pts',(0.696247955557281,2.27861274755843,-0.610312617483778));
#35038=CARTESIAN_POINT('Ctrl Pts',(0.823466790742394,1.74582756814582,1.5867604881466));
#35039=CARTESIAN_POINT('Ctrl Pts',(0.950685625927508,-0.389922248616644,
2.3264200256635));
#35040=CARTESIAN_POINT('Ctrl Pts',(1.07790446111262,-2.16757287041851,0.930806287755246));
#35041=CARTESIAN_POINT('Ctrl Pts',(1.20512329629774,-1.95545520271826,-1.31949954838954));
#35042=CARTESIAN_POINT('Ctrl Pts',(1.33234213148285,0.0518230335398809,
-2.35838898816837));
#35043=CARTESIAN_POINT('Ctrl Pts',(1.45956096666796,2.01150629183162,-1.23231849254524));
#35044=CARTESIAN_POINT('Ctrl Pts',(1.58677980185307,2.12462519346728,1.02505732471468));
#35045=CARTESIAN_POINT('Ctrl Pts',(1.71399863703819,0.287318761604926,2.341408965804));
#35046=CARTESIAN_POINT('Ctrl Pts',(1.8412174722233,-1.8137445999142,1.50834000813179));
#35047=CARTESIAN_POINT('Ctrl Pts',(1.96843630740842,-2.24978152620299,-0.709398069659118));
#35048=CARTESIAN_POINT('Ctrl Pts',(2.09565514259353,-0.620502089064916,
-2.27590338356333));
#35049=CARTESIAN_POINT('Ctrl Pts',(2.22287397777864,1.57839809730298,-1.75311364786995));
#35050=CARTESIAN_POINT('Ctrl Pts',(2.35009281296375,2.32832610584676,0.379041259626889));
#35051=CARTESIAN_POINT('Ctrl Pts',(2.47731164814887,0.940822490842265,2.16324281343369));
#35052=CARTESIAN_POINT('Ctrl Pts',(2.60453048333398,-1.31033627345084,1.96155629457787));
#35053=CARTESIAN_POINT('Ctrl Pts',(2.73174931851909,-2.35864750248118,-0.0408174849469316));
#35054=CARTESIAN_POINT('Ctrl Pts',(2.85896815370421,-1.24161073233134,-2.00578545294822));
#35055=CARTESIAN_POINT('Ctrl Pts',(2.98618698888932,1.01505102673121,-2.12930526437765));
#35056=CARTESIAN_POINT('Ctrl Pts',(3.11340582407443,2.34023742749476,-0.298347997134086));
#35057=CARTESIAN_POINT('Ctrl Pts',(3.24062465925955,1.51640407537933,1.80695219210931));
#35058=CARTESIAN_POINT('Ctrl Pts',(3.36784349444466,-0.698217180620254,
2.25257951257453));
#35059=CARTESIAN_POINT('Ctrl Pts',(3.49506232962978,-2.27434460912666,0.632031074066706));
#35060=CARTESIAN_POINT('Ctrl Pts',(3.62228116481489,-1.7576911784917,-1.57218661975746));
#35061=CARTESIAN_POINT('Ctrl Pts',(3.70709372160496,-0.344875555534673,
-2.07399924429869));
#35062=CARTESIAN_POINT('Ctrl Pts',(3.7495,0.311349471200418,-1.97030177112117));
#35063=CARTESIAN_POINT('Ctrl Pts',(0.275081743211219,-0.941790067967391,
1.92904360906014));
#35064=CARTESIAN_POINT('Ctrl Pts',(0.317488021606256,-1.58427372832989,
1.61537276858829));
#35065=CARTESIAN_POINT('Ctrl Pts',(0.402300578396332,-2.51992744547999,
0.300899277314577));
#35066=CARTESIAN_POINT('Ctrl Pts',(0.529519413581445,-1.61472172164465,
-1.96107696748283));
#35067=CARTESIAN_POINT('Ctrl Pts',(0.656738248766559,0.775007876324146,
-2.41668555342406));
#35068=CARTESIAN_POINT('Ctrl Pts',(0.783957083951671,2.45214790396061,-0.656792957612989));
#35069=CARTESIAN_POINT('Ctrl Pts',(0.911175919136786,1.8787867383313,1.70760538808775));
#35070=CARTESIAN_POINT('Ctrl Pts',(1.0383947543219,-0.419618044214592,2.50359610064302));
#35071=CARTESIAN_POINT('Ctrl Pts',(1.16561358950701,-2.33265142423783,1.00169486454339));
#35072=CARTESIAN_POINT('Ctrl Pts',(1.29283242469213,-2.1043792464395,-1.41999032320318));
#35073=CARTESIAN_POINT('Ctrl Pts',(1.42005125987724,0.055769785018477,-2.53799976334616));
#35074=CARTESIAN_POINT('Ctrl Pts',(1.54727009506235,2.16469908833949,-1.3261697108228));
#35075=CARTESIAN_POINT('Ctrl Pts',(1.67448893024746,2.2864329274227,1.10312389541923));
#35076=CARTESIAN_POINT('Ctrl Pts',(1.80170776543258,0.309200455317831,2.51972657221502));
#35077=CARTESIAN_POINT('Ctrl Pts',(1.92892660061769,-1.95187621229853,1.62321254164996));
#35078=CARTESIAN_POINT('Ctrl Pts',(2.0561454358028,-2.42112094727782,-0.763424584301242));
#35079=CARTESIAN_POINT('Ctrl Pts',(2.18336427098792,-0.667758441505294,
-2.44923219954846));
#35080=CARTESIAN_POINT('Ctrl Pts',(2.31058310617303,1.69860613220222,-1.88662771312737));
#35081=CARTESIAN_POINT('Ctrl Pts',(2.43780194135814,2.50564734455498,0.407908378158857));
#35082=CARTESIAN_POINT('Ctrl Pts',(2.56502077654326,1.0124738841165,2.32799159769612));
#35083=CARTESIAN_POINT('Ctrl Pts',(2.69223961172837,-1.41012918929246,2.11094498677051));
#35084=CARTESIAN_POINT('Ctrl Pts',(2.81945844691349,-2.53827796565631,-0.0439260731183047));
#35085=CARTESIAN_POINT('Ctrl Pts',(2.9466772820986,-1.33616963131785,-2.15854256038544));
#35086=CARTESIAN_POINT('Ctrl Pts',(3.07389611728371,1.09235553530501,-2.29146942433756));
#35087=CARTESIAN_POINT('Ctrl Pts',(3.20111495246883,2.51846581159982,-0.321069658109792));
#35088=CARTESIAN_POINT('Ctrl Pts',(3.32833378765394,1.63189075413675,1.94456650661051));
#35089=CARTESIAN_POINT('Ctrl Pts',(3.45555262283905,-0.751392178333865,
2.4241320233914));
#35090=CARTESIAN_POINT('Ctrl Pts',(3.58277145802416,-2.44755471158052,0.680165453814528));
#35091=CARTESIAN_POINT('Ctrl Pts',(3.70999029320928,-1.89155386046481,-1.69192159940477));
#35092=CARTESIAN_POINT('Ctrl Pts',(3.79480284999935,-0.371140673876142,
-2.23195139462481));
#35093=CARTESIAN_POINT('Ctrl Pts',(3.83720912839439,0.335061301672003,-2.12035650349172));
#35094=CARTESIAN_POINT('Ctrl Pts',(0.362790871605609,-1.00843926415934,
2.06555938931311));
#35095=CARTESIAN_POINT('Ctrl Pts',(0.405197150000647,-1.6963906152377,1.72969049207961));
#35096=CARTESIAN_POINT('Ctrl Pts',(0.490009706790723,-2.69825926741749,
0.322193508003416));
#35097=CARTESIAN_POINT('Ctrl Pts',(0.617228541975836,-1.7289933714334,-2.09985970473909));
#35098=CARTESIAN_POINT('Ctrl Pts',(0.744447377160949,0.82985412471463,-2.58771108773664));
#35099=CARTESIAN_POINT('Ctrl Pts',(0.871666212346062,2.62568306036279,-0.7032732977422));
#35100=CARTESIAN_POINT('Ctrl Pts',(0.998885047531176,2.01174590851678,1.82845028802889));
#35101=CARTESIAN_POINT('Ctrl Pts',(1.12610388271629,-0.449313839812542,
2.68077217562253));
#35102=CARTESIAN_POINT('Ctrl Pts',(1.2533227179014,-2.49772997805715,1.07258344133154));
#35103=CARTESIAN_POINT('Ctrl Pts',(1.38054155308652,-2.25330329016074,-1.52048109801682));
#35104=CARTESIAN_POINT('Ctrl Pts',(1.50776038827163,0.0597165364970737,
-2.71761053852396));
#35105=CARTESIAN_POINT('Ctrl Pts',(1.63497922345674,2.31789188484737,-1.42002092910036));
#35106=CARTESIAN_POINT('Ctrl Pts',(1.76219805864185,2.44824066137811,1.18119046612379));
#35107=CARTESIAN_POINT('Ctrl Pts',(1.88941689382697,0.331082149030738,2.69804417862604));
#35108=CARTESIAN_POINT('Ctrl Pts',(2.01663572901208,-2.09000782468285,1.73808507516812));
#35109=CARTESIAN_POINT('Ctrl Pts',(2.14385456419719,-2.59246036835264,-0.817451098943368));
#35110=CARTESIAN_POINT('Ctrl Pts',(2.27107339938231,-0.715014793945677,
-2.62256101553358));
#35111=CARTESIAN_POINT('Ctrl Pts',(2.39829223456742,1.81881416710148,-2.02014177838479));
#35112=CARTESIAN_POINT('Ctrl Pts',(2.52551106975254,2.6829685832632,0.436775496690829));
#35113=CARTESIAN_POINT('Ctrl Pts',(2.65272990493765,1.08412527739075,2.49274038195854));
#35114=CARTESIAN_POINT('Ctrl Pts',(2.77994874012277,-1.50992210513408,2.26033367896316));
#35115=CARTESIAN_POINT('Ctrl Pts',(2.90716757530787,-2.71790842883145,-0.0470346612896804));
#35116=CARTESIAN_POINT('Ctrl Pts',(3.03438641049299,-1.43072853030436,-2.31129966782265));
#35117=CARTESIAN_POINT('Ctrl Pts',(3.1616052456781,1.1696600438788,-2.45363358429747));
#35118=CARTESIAN_POINT('Ctrl Pts',(3.28882408086321,2.69669419570489,-0.343791319085499));
#35119=CARTESIAN_POINT('Ctrl Pts',(3.41604291604833,1.74737743289418,2.08218082111171));
#35120=CARTESIAN_POINT('Ctrl Pts',(3.54326175123344,-0.804567176047475,
2.59568453420827));
#35121=CARTESIAN_POINT('Ctrl Pts',(3.67048058641855,-2.62076481403437,0.72829983356235));
#35122=CARTESIAN_POINT('Ctrl Pts',(3.79769942160367,-2.02541654243792,-1.81165657905209));
#35123=CARTESIAN_POINT('Ctrl Pts',(3.88251197839374,-0.39740579221761,-2.38990354495094));
#35124=CARTESIAN_POINT('Ctrl Pts',(3.92491825678878,0.358773132143588,-2.27041123586227));
#35125=CARTESIAN_POINT('Ctrl Pts',(0.4505,-1.07508846035128,2.20207516956609));
#35126=CARTESIAN_POINT('Ctrl Pts',(0.492906278395038,-1.80850750214552,
1.84400821557094));
#35127=CARTESIAN_POINT('Ctrl Pts',(0.577718835185112,-2.87659108935499,
0.343487738692257));
#35128=CARTESIAN_POINT('Ctrl Pts',(0.704937670370228,-1.84326502122216,
-2.23864244199535));
#35129=CARTESIAN_POINT('Ctrl Pts',(0.832156505555339,0.884700373105116,
-2.75873662204922));
#35130=CARTESIAN_POINT('Ctrl Pts',(0.959375340740454,2.79921821676497,-0.749753637871415));
#35131=CARTESIAN_POINT('Ctrl Pts',(1.08659417592557,2.14470507870227,1.94929518797004));
#35132=CARTESIAN_POINT('Ctrl Pts',(1.21381301111068,-0.479009635410491,
2.85794825060204));
#35133=CARTESIAN_POINT('Ctrl Pts',(1.34103184629579,-2.66280853187646,1.14347201811968));
#35134=CARTESIAN_POINT('Ctrl Pts',(1.46825068148091,-2.40222733388198,-1.62097187283046));
#35135=CARTESIAN_POINT('Ctrl Pts',(1.59546951666602,0.063663287975671,-2.89722131370176));
#35136=CARTESIAN_POINT('Ctrl Pts',(1.72268835185113,2.47108468135524,-1.51387214737792));
#35137=CARTESIAN_POINT('Ctrl Pts',(1.84990718703624,2.61004839533353,1.25925703682834));
#35138=CARTESIAN_POINT('Ctrl Pts',(1.97712602222136,0.352963842743642,2.87636178503707));
#35139=CARTESIAN_POINT('Ctrl Pts',(2.10434485740647,-2.22813943706718,1.85295760868628));
#35140=CARTESIAN_POINT('Ctrl Pts',(2.23156369259159,-2.76379978942746,-0.871477613585491));
#35141=CARTESIAN_POINT('Ctrl Pts',(2.3587825277767,-0.762271146386054,-2.79588983151871));
#35142=CARTESIAN_POINT('Ctrl Pts',(2.48600136296182,1.93902220200072,-2.15365584364221));
#35143=CARTESIAN_POINT('Ctrl Pts',(2.61322019814693,2.86028982197142,0.4656426152228));
#35144=CARTESIAN_POINT('Ctrl Pts',(2.74043903333204,1.15577667066498,2.65748916622096));
#35145=CARTESIAN_POINT('Ctrl Pts',(2.86765786851715,-1.60971502097569,2.40972237115582));
#35146=CARTESIAN_POINT('Ctrl Pts',(2.99487670370227,-2.89753889200658,-0.050143249461057));
#35147=CARTESIAN_POINT('Ctrl Pts',(3.12209553888738,-1.52528742929087,-2.46405677525986));
#35148=CARTESIAN_POINT('Ctrl Pts',(3.2493143740725,1.2469645524526,-2.61579774425739));
#35149=CARTESIAN_POINT('Ctrl Pts',(3.3765332092576,2.87492257980995,-0.366512980061205));
#35150=CARTESIAN_POINT('Ctrl Pts',(3.50375204444272,1.86286411165161,2.21979513561292));
#35151=CARTESIAN_POINT('Ctrl Pts',(3.63097087962783,-0.857742173761087,
2.76723704502514));
#35152=CARTESIAN_POINT('Ctrl Pts',(3.75818971481295,-2.79397491648822,0.776434213310176));
#35153=CARTESIAN_POINT('Ctrl Pts',(3.88540854999806,-2.15927922441104,-1.93139155869941));
#35154=CARTESIAN_POINT('Ctrl Pts',(3.97022110678813,-0.423670910559079,
-2.54785569527707));
#35155=CARTESIAN_POINT('Ctrl Pts',(4.01262738518317,0.382484962615173,-2.42046596823283));
#35156=CARTESIAN_POINT('Ctrl Pts',(2.99267250378795,-2.45452615968528,-0.000257956296186217));
#35157=CARTESIAN_POINT('Ctrl Pts',(2.99340723709272,-2.45454751304904,-0.0143344873317633));
#35158=CARTESIAN_POINT('Ctrl Pts',(2.99414197039749,-2.45443680249629,-0.0284106766992283));
#35159=CARTESIAN_POINT('Ctrl Pts',(2.99487670370227,-2.45419300304882,-0.0424845669913881));
#35160=CARTESIAN_POINT('Ctrl Pts',(3.0372829820973,-2.44012173776801,-0.854781091393998));
#35161=CARTESIAN_POINT('Ctrl Pts',(3.07968926049234,-1.98270458352944,-1.65941893332693));
#35162=CARTESIAN_POINT('Ctrl Pts',(3.12209553888738,-1.29195400945291,-2.08702801579298));
#35163=CARTESIAN_POINT('Ctrl Pts',(3.16450181728242,-0.601203435376382,
-2.51463709825904));
#35164=CARTESIAN_POINT('Ctrl Pts',(3.20690809567746,0.322880558538104,-2.56521742125821));
#35165=CARTESIAN_POINT('Ctrl Pts',(3.24931437407249,1.05624889338824,-2.21562678872511));
#35166=CARTESIAN_POINT('Ctrl Pts',(3.29172065246753,1.78961722823838,-1.866036156192));
#35167=CARTESIAN_POINT('Ctrl Pts',(3.33412693086257,2.33226990402417,-1.1162745681266));
#35168=CARTESIAN_POINT('Ctrl Pts',(3.37653320925761,2.43491983055733,-0.310342421481551));
#35169=CARTESIAN_POINT('Ctrl Pts',(3.41893948765264,2.5375697570905,0.495589725163502));
#35170=CARTESIAN_POINT('Ctrl Pts',(3.46134576604768,2.20021693437105,1.35769243038821));
#35171=CARTESIAN_POINT('Ctrl Pts',(3.50375204444272,1.57810614210921,1.87998410123594));
#35172=CARTESIAN_POINT('Ctrl Pts',(3.54615832283776,0.955995349847373,2.40227577208366));
#35173=CARTESIAN_POINT('Ctrl Pts',(3.58856460123279,0.0491265880431435,
2.5847564085544));
#35174=CARTESIAN_POINT('Ctrl Pts',(3.63097087962783,-0.727013249980161,
2.34419625483728));
#35175=CARTESIAN_POINT('Ctrl Pts',(3.67048058641855,-1.45013865945934,2.1200676234503));
#35176=CARTESIAN_POINT('Ctrl Pts',(3.70999029320928,-2.05978415989638,1.52871627651428));
#35177=CARTESIAN_POINT('Ctrl Pts',(3.7495,-2.31513335459632,0.815631492636623));
#35178=CARTESIAN_POINT('',(0.4505,-1.16034898466907,-1.62253437445173));
#35179=CARTESIAN_POINT('Ctrl Pts',(0.450499999999999,-1.16286240980301,
-1.62484720205836));
#35180=CARTESIAN_POINT('Ctrl Pts',(0.450499999999999,-1.20286330961462,
-1.60271479777366));
#35181=CARTESIAN_POINT('Ctrl Pts',(0.450499999999999,-1.24197977006801,
-1.579152801667));
#35182=CARTESIAN_POINT('Ctrl Pts',(0.450499999999999,-1.28012567116714,
-1.55417759699536));
#35183=CARTESIAN_POINT('Ctrl Pts',(0.4505,-1.34003952566005,-1.5149502950963));
#35184=CARTESIAN_POINT('Ctrl Pts',(0.4505,-1.39756042503822,-1.47223942604334));
#35185=CARTESIAN_POINT('Ctrl Pts',(0.4505,-1.45260638718602,-1.42638958840563));
#35186=CARTESIAN_POINT('Ctrl Pts',(0.450499999999999,-1.48312159761652,
-1.40097233000688));
#35187=CARTESIAN_POINT('Ctrl Pts',(0.4505,-1.51287592931269,-1.37458951272792));
#35188=CARTESIAN_POINT('Ctrl Pts',(0.4505,-1.54185269550254,-1.34729371270681));
#35189=CARTESIAN_POINT('Ctrl Pts',(0.4505,-1.55613672552596,-1.3338383110771));
#35190=CARTESIAN_POINT('Ctrl Pts',(0.4505,-1.57023177572244,-1.32016099482662));
#35191=CARTESIAN_POINT('Ctrl Pts',(0.4505,-1.58413563760341,-1.30626771878357));
#35192=CARTESIAN_POINT('Ctrl Pts',(0.4505,-1.59424325015721,-1.29616780175704));
#35193=CARTESIAN_POINT('Ctrl Pts',(0.4505,-1.60424293841027,-1.2859606250128));
#35194=CARTESIAN_POINT('Ctrl Pts',(0.4505,-1.61413396809427,-1.27564913736583));
#35195=CARTESIAN_POINT('Ctrl Pts',(0.4505,-1.66618304361349,-1.22138750673695));
#35196=CARTESIAN_POINT('Ctrl Pts',(0.4505,-1.71522672419473,-1.16423977664219));
#35197=CARTESIAN_POINT('Ctrl Pts',(0.4505,-1.76117091050649,-1.10457870598492));
#35198=CARTESIAN_POINT('Ctrl Pts',(0.4505,-1.79851739430398,-1.05608222824728));
#35199=CARTESIAN_POINT('Ctrl Pts',(0.4505,-1.83381563167038,-1.00592385645458));
#35200=CARTESIAN_POINT('Ctrl Pts',(0.4505,-1.86700175841926,-0.954282216791985));
#35201=CARTESIAN_POINT('Ctrl Pts',(0.4505,-1.8801338745443,-0.933847050794197));
#35202=CARTESIAN_POINT('Ctrl Pts',(0.4505,-1.8929351120508,-0.913179436076022));
#35203=CARTESIAN_POINT('Ctrl Pts',(0.4505,-1.90540088753822,-0.892289759695898));
#35204=CARTESIAN_POINT('Ctrl Pts',(0.4505,-1.91424907112747,-0.877462307371091));
#35205=CARTESIAN_POINT('Ctrl Pts',(0.4505,-1.92292961817841,-0.86252027332416));
#35206=CARTESIAN_POINT('Ctrl Pts',(0.4505,-1.93142873757601,-0.847489309628046));
#35207=CARTESIAN_POINT('Ctrl Pts',(0.4505,-1.96971919482744,-0.779771414875745));
#35208=CARTESIAN_POINT('Ctrl Pts',(0.4505,-2.00438315634146,-0.710165083960324));
#35209=CARTESIAN_POINT('Ctrl Pts',(0.4505,-2.0353241077575,-0.639048694689319));
#35210=CARTESIAN_POINT('Ctrl Pts',(0.4505,-2.06685107805879,-0.566585367290814));
#35211=CARTESIAN_POINT('Ctrl Pts',(0.4505,-2.09451336057944,-0.49255347892645));
#35212=CARTESIAN_POINT('Ctrl Pts',(0.4505,-2.11817370236006,-0.417312725162707));
#35213=CARTESIAN_POINT('Ctrl Pts',(0.4505,-2.13546259495292,-0.362333413262279));
#35214=CARTESIAN_POINT('Ctrl Pts',(0.4505,-2.15061399663607,-0.30670773008184));
#35215=CARTESIAN_POINT('Ctrl Pts',(0.4505,-2.16355960203642,-0.250566432797886));
#35216=CARTESIAN_POINT('Ctrl Pts',(0.4505,-2.17326880608668,-0.20846045983492));
#35217=CARTESIAN_POINT('Ctrl Pts',(0.4505,-2.18173700276312,-0.1660642755761));
#35218=CARTESIAN_POINT('Ctrl Pts',(0.4505,-2.18893003555588,-0.123431179597991));
#35219=CARTESIAN_POINT('Ctrl Pts',(0.4505,-2.19111103153329,-0.110504419285397));
#35220=CARTESIAN_POINT('Ctrl Pts',(0.4505,-2.19317506525113,-0.0975538196791666));
#35221=CARTESIAN_POINT('Ctrl Pts',(0.4505,-2.19512011992499,-0.0845873892082416));
#35222=CARTESIAN_POINT('Ctrl Pts',(0.4505,-2.2071501360141,-0.00439099715827403));
#35223=CARTESIAN_POINT('Ctrl Pts',(0.4505,-2.21459346758939,0.0761401520900184));
#35224=CARTESIAN_POINT('Ctrl Pts',(0.4505,-2.21732325800404,0.15662739588242));
#35225=CARTESIAN_POINT('Ctrl Pts',(0.4505,-2.2185190065568,0.191883767494183));
#35226=CARTESIAN_POINT('Ctrl Pts',(0.4505,-2.21880979474632,0.227132116865632));
#35227=CARTESIAN_POINT('Ctrl Pts',(0.4505,-2.21818221942756,0.262342172420224));
#35228=CARTESIAN_POINT('Ctrl Pts',(0.4505,-2.21679935655232,0.339927566884592));
#35229=CARTESIAN_POINT('Ctrl Pts',(0.4505,-2.21096111363732,0.41732659146968));
#35230=CARTESIAN_POINT('Ctrl Pts',(0.4505,-2.20090098242755,0.49428846405244));
#35231=CARTESIAN_POINT('Ctrl Pts',(0.4505,-2.19063003840118,0.572863093843948));
#35232=CARTESIAN_POINT('Ctrl Pts',(0.4505,-2.17595829487236,0.65098282970126));
#35233=CARTESIAN_POINT('Ctrl Pts',(0.4505,-2.15708029963991,0.728383125138283));
#35234=CARTESIAN_POINT('Ctrl Pts',(0.4505,-2.15396392646031,0.741160340188063));
#35235=CARTESIAN_POINT('Ctrl Pts',(0.4505,-2.15073281306651,0.753917939175734));
#35236=CARTESIAN_POINT('Ctrl Pts',(0.4505,-2.14738770094255,0.766654714405889));
#35237=CARTESIAN_POINT('Ctrl Pts',(0.4505,-2.1442095939825,0.778755604453134));
#35238=CARTESIAN_POINT('Ctrl Pts',(0.4505,-2.14093109831446,0.790828124513886));
#35239=CARTESIAN_POINT('Ctrl Pts',(0.4505,-2.13755345581554,0.802870818443932));
#35240=CARTESIAN_POINT('Ctrl Pts',(0.4505,-2.11567321858042,0.880882923106774));
#35241=CARTESIAN_POINT('Ctrl Pts',(0.4505,-2.0896352327598,0.957648854289395));
#35242=CARTESIAN_POINT('Ctrl Pts',(0.4505,-2.05971373326038,1.03289773290721));
#35243=CARTESIAN_POINT('Ctrl Pts',(0.4505,-2.02920890208329,1.10961361870521));
#35244=CARTESIAN_POINT('Ctrl Pts',(0.4505,-1.99466746728849,1.18475355617105));
#35245=CARTESIAN_POINT('Ctrl Pts',(0.4505,-1.95632475170503,1.25803177794143));
#35246=CARTESIAN_POINT('Ctrl Pts',(0.4505,-1.91771233699759,1.33182543196321));
#35247=CARTESIAN_POINT('Ctrl Pts',(0.4505,-1.8752446472627,1.40373200500635));
#35248=CARTESIAN_POINT('Ctrl Pts',(0.4505,-1.8291106405353,1.47344764264672));
#35249=CARTESIAN_POINT('Ctrl Pts',(0.4505,-1.81079706334026,1.50112229746639));
#35250=CARTESIAN_POINT('Ctrl Pts',(0.4505,-1.79190520610228,1.52845149410343));
#35251=CARTESIAN_POINT('Ctrl Pts',(0.4505,-1.77244484874189,1.55541520292446));
#35252=CARTESIAN_POINT('Ctrl Pts',(0.4505,-1.76269243849393,1.56892786075285));
#35253=CARTESIAN_POINT('Ctrl Pts',(0.4505,-1.75279510256798,1.58235137285538));
#35254=CARTESIAN_POINT('Ctrl Pts',(0.4505,-1.74276980623577,1.59566264979496));
#35255=CARTESIAN_POINT('Ctrl Pts',(0.4505,-1.69110824500774,1.66425726544013));
#35256=CARTESIAN_POINT('Ctrl Pts',(0.4505,-1.63597635124539,1.72998168578403));
#35257=CARTESIAN_POINT('Ctrl Pts',(0.4505,-1.57763057533434,1.79253936164174));
#35258=CARTESIAN_POINT('Ctrl Pts',(0.4505,-1.51919556506657,1.85519271355955));
#35259=CARTESIAN_POINT('Ctrl Pts',(0.4505,-1.45753640083401,1.9146705632344));
#35260=CARTESIAN_POINT('Ctrl Pts',(0.4505,-1.39286151373016,1.9706576018754));
#35261=CARTESIAN_POINT('Ctrl Pts',(0.4505,-1.32955892208391,2.02545668701153));
#35262=CARTESIAN_POINT('Ctrl Pts',(0.4505,-1.26336666868825,2.07691231275167));
#35263=CARTESIAN_POINT('Ctrl Pts',(0.4505,-1.19444070240512,2.1246995984667));
#35264=CARTESIAN_POINT('Ctrl Pts',(0.4505,-1.15552113289993,2.15168305170129));
#35265=CARTESIAN_POINT('Ctrl Pts',(0.4505,-1.11572927824821,2.17749630300684));
#35266=CARTESIAN_POINT('Ctrl Pts',(0.4505,-1.07508846035128,2.20207516956609));
#35267=CARTESIAN_POINT('Ctrl Pts',(0.4505,-1.162862409803,-1.62484720205837));
#35268=CARTESIAN_POINT('Ctrl Pts',(0.490009706790723,-0.659641438489814,
-1.98109404025392));
#35269=CARTESIAN_POINT('Ctrl Pts',(0.571925691976483,0.755645094302849,
-2.20842574605865));
#35270=CARTESIAN_POINT('Ctrl Pts',(0.696247955557281,2.27861274755843,-0.610312617483778));
#35271=CARTESIAN_POINT('Ctrl Pts',(0.823466790742394,1.74582756814582,1.5867604881466));
#35272=CARTESIAN_POINT('Ctrl Pts',(0.950685625927508,-0.389922248616644,
2.3264200256635));
#35273=CARTESIAN_POINT('Ctrl Pts',(1.05271173521497,-1.81555058699103,1.20717506842332));
#35274=CARTESIAN_POINT('Ctrl Pts',(1.11233156610739,-1.99312914321941,0.271569088097866));
#35275=CARTESIAN_POINT('Ctrl Pts',(1.12954511860477,-1.99192664249562,0.000999255222959156));
#35276=CARTESIAN_POINT('Origin',(0.4505,-5.69858952725515E-16,8.58067791224701E-17));
#35277=CARTESIAN_POINT('',(0.4505,-2.4505,-3.00099698131059E-16));
#35278=CARTESIAN_POINT('Origin',(0.4505,0.,0.));
#35279=CARTESIAN_POINT('Origin',(0.4505,0.,0.));
#35280=CARTESIAN_POINT('',(0.4505,1.16034898466907,-1.62253437445173));
#35281=CARTESIAN_POINT('Ctrl Pts',(0.4505,1.07766119456972,2.20539011734829));
#35282=CARTESIAN_POINT('Ctrl Pts',(0.4505,1.1253722485115,2.17681124103074));
#35283=CARTESIAN_POINT('Ctrl Pts',(0.450499999999999,1.17197132590231,2.14653322621614));
#35284=CARTESIAN_POINT('Ctrl Pts',(0.450499999999999,1.21735566783477,2.11455018800921));
#35285=CARTESIAN_POINT('Ctrl Pts',(0.450499999999999,1.28700221983055,2.06546920019237));
#35286=CARTESIAN_POINT('Ctrl Pts',(0.4505,1.35379019187679,2.01237416511058));
#35287=CARTESIAN_POINT('Ctrl Pts',(0.4505,1.41755123156995,1.95562691189186));
#35288=CARTESIAN_POINT('Ctrl Pts',(0.4505,1.44984247863091,1.9268877385262));
#35289=CARTESIAN_POINT('Ctrl Pts',(0.450499999999999,1.48135671953801,1.89721129791422));
#35290=CARTESIAN_POINT('Ctrl Pts',(0.450499999999999,1.51206782367031,1.86664196767908));
#35291=CARTESIAN_POINT('Ctrl Pts',(0.450499999999999,1.53122947677371,1.8475687719045));
#35292=CARTESIAN_POINT('Ctrl Pts',(0.450499999999999,1.5500784167829,1.82814795145982));
#35293=CARTESIAN_POINT('Ctrl Pts',(0.450499999999999,1.56860768548358,1.80839005248937));
#35294=CARTESIAN_POINT('Ctrl Pts',(0.450499999999999,1.58037795787674,1.7958393222606));
#35295=CARTESIAN_POINT('Ctrl Pts',(0.450499999999999,1.59201302261345,1.78315914283905));
#35296=CARTESIAN_POINT('Ctrl Pts',(0.450499999999999,1.60350833805641,1.77035617908208));
#35297=CARTESIAN_POINT('Ctrl Pts',(0.450499999999999,1.660267874257,1.70713996823124));
#35298=CARTESIAN_POINT('Ctrl Pts',(0.4505,1.71365006389022,1.64090458616163));
#35299=CARTESIAN_POINT('Ctrl Pts',(0.4505,1.7634832017426,1.57200692669245));
#35300=CARTESIAN_POINT('Ctrl Pts',(0.4505,1.80175234668051,1.51909726397123));
#35301=CARTESIAN_POINT('Ctrl Pts',(0.450499999999999,1.83792764492218,1.46461675962789));
#35302=CARTESIAN_POINT('Ctrl Pts',(0.450499999999999,1.87191183530092,1.40871961920951));
#35303=CARTESIAN_POINT('Ctrl Pts',(0.450499999999999,1.88877785857892,1.38097841187271));
#35304=CARTESIAN_POINT('Ctrl Pts',(0.450499999999999,1.90510392941073,1.35288821271951));
#35305=CARTESIAN_POINT('Ctrl Pts',(0.450499999999999,1.92087647850637,1.32446762860519));
#35306=CARTESIAN_POINT('Ctrl Pts',(0.4505,1.9303350350449,1.30742423884786));
#35307=CARTESIAN_POINT('Ctrl Pts',(0.4505,1.93959678388073,1.29025743573171));
#35308=CARTESIAN_POINT('Ctrl Pts',(0.4505,1.94864464124469,1.27299863809729));
#35309=CARTESIAN_POINT('Ctrl Pts',(0.4505,1.98726093032314,1.19933802522641));
#35310=CARTESIAN_POINT('Ctrl Pts',(0.450499999999999,2.02203257416733,1.12392171655336));
#35311=CARTESIAN_POINT('Ctrl Pts',(0.450499999999999,2.05279909002309,1.04708127458096));
#35312=CARTESIAN_POINT('Ctrl Pts',(0.4505,2.08291604831929,0.971863125174856));
#35313=CARTESIAN_POINT('Ctrl Pts',(0.450499999999999,2.10919534613456,0.895279401798556));
#35314=CARTESIAN_POINT('Ctrl Pts',(0.450499999999999,2.13143843939754,0.817632103176601));
#35315=CARTESIAN_POINT('Ctrl Pts',(0.4505,2.15319308716667,0.74168989443012));
#35316=CARTESIAN_POINT('Ctrl Pts',(0.4505,2.17108694519009,0.664729532655734));
#35317=CARTESIAN_POINT('Ctrl Pts',(0.4505,2.18488617170524,0.587037321507561));
#35318=CARTESIAN_POINT('Ctrl Pts',(0.4505,2.18972785922178,0.559777720512106));
#35319=CARTESIAN_POINT('Ctrl Pts',(0.4505,2.19406502052564,0.532428111547084));
#35320=CARTESIAN_POINT('Ctrl Pts',(0.4505,2.19788607277123,0.505001239804802));
#35321=CARTESIAN_POINT('Ctrl Pts',(0.4505,2.20008575405405,0.489212296723147));
#35322=CARTESIAN_POINT('Ctrl Pts',(0.450499999999999,2.2021143818284,0.473397753261568));
#35323=CARTESIAN_POINT('Ctrl Pts',(0.450499999999999,2.2039696260404,0.457560083389685));
#35324=CARTESIAN_POINT('Ctrl Pts',(0.450499999999999,2.20542249242619,0.445157393739837));
#35325=CARTESIAN_POINT('Ctrl Pts',(0.4505,2.20676796699628,0.432749475626273));
#35326=CARTESIAN_POINT('Ctrl Pts',(0.4505,2.20800521290325,0.420339348883872));
#35327=CARTESIAN_POINT('Ctrl Pts',(0.4505,2.21574988769131,0.342656816125777));
#35328=CARTESIAN_POINT('Ctrl Pts',(0.4505,2.2192608461013,0.264863324756902));
#35329=CARTESIAN_POINT('Ctrl Pts',(0.4505,2.21835792731929,0.187237833426566));
#35330=CARTESIAN_POINT('Ctrl Pts',(0.4505,2.21805232660199,0.160964810531994));
#35331=CARTESIAN_POINT('Ctrl Pts',(0.4505,2.21724066358271,0.13471106740812));
#35332=CARTESIAN_POINT('Ctrl Pts',(0.4505,2.21591459644172,0.108487611054857));
#35333=CARTESIAN_POINT('Ctrl Pts',(0.4505,2.21191623246908,0.029418520298201));
#35334=CARTESIAN_POINT('Ctrl Pts',(0.4505,2.20324469891092,-0.0493767922785765));
#35335=CARTESIAN_POINT('Ctrl Pts',(0.4505,2.19008710614742,-0.127579539719568));
#35336=CARTESIAN_POINT('Ctrl Pts',(0.4505,2.17718423010061,-0.204268366839285));
#35337=CARTESIAN_POINT('Ctrl Pts',(0.450499999999999,2.15996657536957,-0.280388073854071));
#35338=CARTESIAN_POINT('Ctrl Pts',(0.450499999999999,2.13857057363323,-0.355611797093477));
#35339=CARTESIAN_POINT('Ctrl Pts',(0.450499999999999,2.13331188408938,-0.374100214309137));
#35340=CARTESIAN_POINT('Ctrl Pts',(0.4505,2.12779838008763,-0.392541028423528));
#35341=CARTESIAN_POINT('Ctrl Pts',(0.4505,2.12204347435241,-0.410893253784562));
#35342=CARTESIAN_POINT('Ctrl Pts',(0.4505,2.09876348753168,-0.485132447994281));
#35343=CARTESIAN_POINT('Ctrl Pts',(0.4505,2.0715155754429,-0.558010645131724));
#35344=CARTESIAN_POINT('Ctrl Pts',(0.4505,2.0405037686822,-0.629236342323922));
#35345=CARTESIAN_POINT('Ctrl Pts',(0.4505,2.00952043889923,-0.700396635632768));
#35346=CARTESIAN_POINT('Ctrl Pts',(0.4505,1.97477945052421,-0.769908288945355));
#35347=CARTESIAN_POINT('Ctrl Pts',(0.4505,1.93644161811572,-0.837451348638747));
#35348=CARTESIAN_POINT('Ctrl Pts',(0.4505,1.89874831846993,-0.903858879479057));
#35349=CARTESIAN_POINT('Ctrl Pts',(0.4505,1.85757740508633,-0.968364102521197));
#35350=CARTESIAN_POINT('Ctrl Pts',(0.4505,1.81305071976513,-1.0306238622284));
#35351=CARTESIAN_POINT('Ctrl Pts',(0.4505,1.79614454072544,-1.05426304931329));
#35352=CARTESIAN_POINT('Ctrl Pts',(0.4505,1.77875431794757,-1.07757806955031));
#35353=CARTESIAN_POINT('Ctrl Pts',(0.4505,1.76088583128245,-1.10054833472365));
#35354=CARTESIAN_POINT('Ctrl Pts',(0.4505,1.75326867502042,-1.11034032788372));
#35355=CARTESIAN_POINT('Ctrl Pts',(0.4505,1.74556442525531,-1.1200697467296));
#35356=CARTESIAN_POINT('Ctrl Pts',(0.4505,1.73778290495544,-1.12972366725519));
#35357=CARTESIAN_POINT('Ctrl Pts',(0.4505,1.69071713631285,-1.18811446653882));
#35358=CARTESIAN_POINT('Ctrl Pts',(0.4505,1.64074593468803,-1.24385231590744));
#35359=CARTESIAN_POINT('Ctrl Pts',(0.4505,1.58802192138046,-1.29665175191528));
#35360=CARTESIAN_POINT('Ctrl Pts',(0.4505,1.53615421651406,-1.34859365451648));
#35361=CARTESIAN_POINT('Ctrl Pts',(0.4505,1.48162173354821,-1.39769237127414));
#35362=CARTESIAN_POINT('Ctrl Pts',(0.4505,1.424543005305,-1.44363421728573));
#35363=CARTESIAN_POINT('Ctrl Pts',(0.4505,1.36929311706813,-1.4881040563249));
#35364=CARTESIAN_POINT('Ctrl Pts',(0.4505,1.31165695283869,-1.52961639546006));
#35365=CARTESIAN_POINT('Ctrl Pts',(0.4505,1.25172579891194,-1.56784107051692));
#35366=CARTESIAN_POINT('Ctrl Pts',(0.4505,1.22183450271092,-1.58690603104995));
#35367=CARTESIAN_POINT('Ctrl Pts',(0.4505,1.19137209683489,-1.60515239365456));
#35368=CARTESIAN_POINT('Ctrl Pts',(0.4505,1.16034898466907,-1.62253437445173));
#35369=CARTESIAN_POINT('Origin',(0.4505,0.,0.));
#35370=CARTESIAN_POINT('Origin',(-1.02854511860477,0.,0.));
#35371=CARTESIAN_POINT('Ctrl Pts',(0.4505,1.16034898466907,-1.62253437445173));
#35372=CARTESIAN_POINT('Ctrl Pts',(0.492906278395038,1.70074725201027,-1.23607070952126));
#35373=CARTESIAN_POINT('Ctrl Pts',(0.577718835185113,2.35553983219541,0.112669531194497));
#35374=CARTESIAN_POINT('Ctrl Pts',(0.704937670370226,1.17739386665123,2.04593681646151));
#35375=CARTESIAN_POINT('Ctrl Pts',(0.83215650555534,-1.0826777789212,2.09509384907487));
#35376=CARTESIAN_POINT('Ctrl Pts',(0.920995575897006,-1.96647049832517,
0.78840734607953));
#35377=CARTESIAN_POINT('Ctrl Pts',(0.967428367843636,-1.99769546358392,
0.0640753932799172));
#35378=CARTESIAN_POINT('Ctrl Pts',(0.971454881395227,-1.99728088898927,
0.00122486924751962));
#35379=CARTESIAN_POINT('Ctrl Pts',(0.187372614816828,1.42545942445497,-1.99324250386964));
#35380=CARTESIAN_POINT('Ctrl Pts',(0.229778893211866,2.08932504877863,-1.51848165117526));
#35381=CARTESIAN_POINT('Ctrl Pts',(0.314591450001941,2.89372119754097,0.138411673739624));
#35382=CARTESIAN_POINT('Ctrl Pts',(0.441810285187055,1.44639863152217,2.51338171136179));
#35383=CARTESIAN_POINT('Ctrl Pts',(0.569029120372167,-1.33004230968612,
2.57376988452587));
#35384=CARTESIAN_POINT('Ctrl Pts',(0.696247955557282,-2.88480482818958,
0.275055317538262));
#35385=CARTESIAN_POINT('Ctrl Pts',(0.823466790742394,-1.79165965660462,
-2.27804038996095));
#35386=CARTESIAN_POINT('Ctrl Pts',(0.950685625927509,0.946429080626742,
-2.73890203154562));
#35387=CARTESIAN_POINT('Ctrl Pts',(1.07790446111262,2.81559143218447,-0.685944933469733));
#35388=CARTESIAN_POINT('Ctrl Pts',(1.20512329629773,2.10007452551338,1.99698045214554));
#35389=CARTESIAN_POINT('Ctrl Pts',(1.33234213148285,-0.54335094423318,2.84652607934227));
#35390=CARTESIAN_POINT('Ctrl Pts',(1.45956096666796,-2.68796270560187,1.08301537658065));
#35391=CARTESIAN_POINT('Ctrl Pts',(1.58677980185308,-2.36501524531905,-1.67474809746095));
#35392=CARTESIAN_POINT('Ctrl Pts',(1.71399863703819,0.129035324547271,-2.89506263077516));
#35393=CARTESIAN_POINT('Ctrl Pts',(1.8412174722233,2.50462795093246,-1.45770139723891));
#35394=CARTESIAN_POINT('Ctrl Pts',(1.96843630740841,2.58095870736468,1.31784367962883));
#35395=CARTESIAN_POINT('Ctrl Pts',(2.09565514259353,0.287949939112121,2.88359833691687));
#35396=CARTESIAN_POINT('Ctrl Pts',(2.22287397777864,-2.26939342905054,1.80219067117606));
#35397=CARTESIAN_POINT('Ctrl Pts',(2.35009281296376,-2.74342899054083,-0.933635728965404));
#35398=CARTESIAN_POINT('Ctrl Pts',(2.47731164814887,-0.698961077714174,
-2.81238674873448));
#35399=CARTESIAN_POINT('Ctrl Pts',(2.60453048333398,1.98712247865483,-2.10933288596168));
#35400=CARTESIAN_POINT('Ctrl Pts',(2.73174931851909,2.84908212195303,0.530070751248655));
#35401=CARTESIAN_POINT('Ctrl Pts',(2.85896815370421,1.09543795124656,2.68292587667123));
#35402=CARTESIAN_POINT('Ctrl Pts',(2.98618698888932,-1.6635791259226,2.3727235057746));
#35403=CARTESIAN_POINT('Ctrl Pts',(3.11340582407443,-2.89589144198292,-0.115434395429308));
#35404=CARTESIAN_POINT('Ctrl Pts',(3.24062465925955,-1.46885379292453,-2.49804380655408));
#35405=CARTESIAN_POINT('Ctrl Pts',(3.36784349444466,1.30486728963842,-2.58662430988328));
#35406=CARTESIAN_POINT('Ctrl Pts',(3.49506232962977,2.88406110179725,-0.302238629855752));
#35407=CARTESIAN_POINT('Ctrl Pts',(3.62228116481489,1.8089990872024,2.26280853432768));
#35408=CARTESIAN_POINT('Ctrl Pts',(3.70709372160496,-0.00481760480854868,
2.58283613012782));
#35409=CARTESIAN_POINT('Ctrl Pts',(3.7495,-0.778675485261984,2.32349192782157));
#35410=CARTESIAN_POINT('Ctrl Pts',(0.275081743211218,1.33708927785967,-1.869673127397));
#35411=CARTESIAN_POINT('Ctrl Pts',(0.317488021606256,1.95979911652251,-1.42434467062392));
#35412=CARTESIAN_POINT('Ctrl Pts',(0.402300578396332,2.71432740909245,0.129830959557915));
#35413=CARTESIAN_POINT('Ctrl Pts',(0.529519413581445,1.35673037656519,2.35756674639503));
#35414=CARTESIAN_POINT('Ctrl Pts',(0.656738248766558,-1.24758746609781,
2.4142112060422));
#35415=CARTESIAN_POINT('Ctrl Pts',(0.783957083951673,-2.7059638024877,0.258003496689719));
#35416=CARTESIAN_POINT('Ctrl Pts',(0.911175919136785,-1.68058723757483,
-2.13681521037519));
#35417=CARTESIAN_POINT('Ctrl Pts',(1.0383947543219,0.887756013430166,-2.56910612582884));
#35418=CARTESIAN_POINT('Ctrl Pts',(1.16561358950701,2.64104123219561,-0.643420359786968));
#35419=CARTESIAN_POINT('Ctrl Pts',(1.29283242469212,1.96988218857497,1.87317934474361));
#35420=CARTESIAN_POINT('Ctrl Pts',(1.42005125987724,-0.509666363829961,
2.67005811217091));
#35421=CARTESIAN_POINT('Ctrl Pts',(1.54727009506235,-2.52132474014202,1.01587475794817));
#35422=CARTESIAN_POINT('Ctrl Pts',(1.67448893024747,-2.21839813342976,-1.57092351126523));
#35423=CARTESIAN_POINT('Ctrl Pts',(1.80170776543258,0.12103588917185,-2.71558568131236));
#35424=CARTESIAN_POINT('Ctrl Pts',(1.92892660061769,2.34935566791029,-1.36733243691902));
#35425=CARTESIAN_POINT('Ctrl Pts',(2.05614543580281,2.42095436391349,1.2361450797525));
#35426=CARTESIAN_POINT('Ctrl Pts',(2.18336427098792,0.270098727148528,2.70483210661695));
#35427=CARTESIAN_POINT('Ctrl Pts',(2.31058310617303,-2.12870431046389,1.69046539084028));
#35428=CARTESIAN_POINT('Ctrl Pts',(2.43780194135815,-2.57335243984519,-0.875755774741645));
#35429=CARTESIAN_POINT('Ctrl Pts',(2.56502077654326,-0.655629579221588,
-2.63803522037486));
#35430=CARTESIAN_POINT('Ctrl Pts',(2.69223961172837,1.86393250794859,-1.97856658482899));
#35431=CARTESIAN_POINT('Ctrl Pts',(2.81945844691348,2.67245569509047,0.497209465132684));
#35432=CARTESIAN_POINT('Ctrl Pts',(2.9466772820986,1.02752720564626,2.51660016514394));
#35433=CARTESIAN_POINT('Ctrl Pts',(3.07389611728371,-1.56044695063331,2.22562852682381));
#35434=CARTESIAN_POINT('Ctrl Pts',(3.20111495246883,-2.71636311107307,-0.108278138105376));
#35435=CARTESIAN_POINT('Ctrl Pts',(3.32833378765393,-1.37779344930413,-2.34317970197175));
#35436=CARTESIAN_POINT('Ctrl Pts',(3.45555262283906,1.22397315004069,-2.42626873221488));
#35437=CARTESIAN_POINT('Ctrl Pts',(3.58277145802416,2.70526618278153,-0.283501602642697));
#35438=CARTESIAN_POINT('Ctrl Pts',(3.70999029320928,1.69685172489641,2.12252764069783));
#35439=CARTESIAN_POINT('Ctrl Pts',(3.79480284999935,-0.00451894148929613,
2.42271539744663));
#35440=CARTESIAN_POINT('Ctrl Pts',(3.83720912839439,-0.730402159762679,
2.17944901874116));
#35441=CARTESIAN_POINT('Ctrl Pts',(0.362790871605609,1.24871913126437,-1.74610375092437));
#35442=CARTESIAN_POINT('Ctrl Pts',(0.405197150000647,1.83027318426639,-1.33020769007259));
#35443=CARTESIAN_POINT('Ctrl Pts',(0.490009706790722,2.53493362064393,0.121250245376206));
#35444=CARTESIAN_POINT('Ctrl Pts',(0.617228541975837,1.26706212160821,2.20175178142827));
#35445=CARTESIAN_POINT('Ctrl Pts',(0.744447377160948,-1.1651326225095,2.25465252755853));
#35446=CARTESIAN_POINT('Ctrl Pts',(0.871666212346063,-2.52712277678581,
0.240951675841176));
#35447=CARTESIAN_POINT('Ctrl Pts',(0.998885047531177,-1.56951481854503,
-1.99559003078943));
#35448=CARTESIAN_POINT('Ctrl Pts',(1.12610388271629,0.829082946233588,-2.39931022011206));
#35449=CARTESIAN_POINT('Ctrl Pts',(1.2533227179014,2.46649103220676,-0.600895786104207));
#35450=CARTESIAN_POINT('Ctrl Pts',(1.38054155308651,1.83968985163656,1.74937823734167));
#35451=CARTESIAN_POINT('Ctrl Pts',(1.50776038827163,-0.475981783426744,
2.49359014499956));
#35452=CARTESIAN_POINT('Ctrl Pts',(1.63497922345674,-2.35468677468218,0.948734139315698));
#35453=CARTESIAN_POINT('Ctrl Pts',(1.76219805864186,-2.07178102154046,-1.46709892506951));
#35454=CARTESIAN_POINT('Ctrl Pts',(1.88941689382697,0.113036453796428,-2.53610873184956));
#35455=CARTESIAN_POINT('Ctrl Pts',(2.01663572901208,2.19408338488812,-1.27696347659914));
#35456=CARTESIAN_POINT('Ctrl Pts',(2.14385456419719,2.26095002046229,1.15444647987618));
#35457=CARTESIAN_POINT('Ctrl Pts',(2.27107339938231,0.252247515184935,2.52606587631703));
#35458=CARTESIAN_POINT('Ctrl Pts',(2.39829223456742,-1.98801519187724,1.5787401105045));
#35459=CARTESIAN_POINT('Ctrl Pts',(2.52551106975254,-2.40327588914955,-0.817875820517883));
#35460=CARTESIAN_POINT('Ctrl Pts',(2.65272990493765,-0.612298080729003,
-2.46368369201524));
#35461=CARTESIAN_POINT('Ctrl Pts',(2.77994874012277,1.74074253724235,-1.84780028369628));
#35462=CARTESIAN_POINT('Ctrl Pts',(2.90716757530787,2.49582926822791,0.464348179016712));
#35463=CARTESIAN_POINT('Ctrl Pts',(3.03438641049299,0.959616460045959,2.35027445361664));
#35464=CARTESIAN_POINT('Ctrl Pts',(3.1616052456781,-1.45731477534402,2.07853354787301));
#35465=CARTESIAN_POINT('Ctrl Pts',(3.28882408086321,-2.53683478016323,-0.101121880781441));
#35466=CARTESIAN_POINT('Ctrl Pts',(3.41604291604833,-1.28673310568374,-2.18831559738942));
#35467=CARTESIAN_POINT('Ctrl Pts',(3.54326175123344,1.14307901044296,-2.26591315454646));
#35468=CARTESIAN_POINT('Ctrl Pts',(3.67048058641856,2.5264712637658,-0.264764575429645));
#35469=CARTESIAN_POINT('Ctrl Pts',(3.79769942160367,1.58470436259042,1.98224674706799));
#35470=CARTESIAN_POINT('Ctrl Pts',(3.88251197839374,-0.00422027817004178,
2.26259466476544));
#35471=CARTESIAN_POINT('Ctrl Pts',(3.92491825678878,-0.682128834263374,
2.03540610966074));
#35472=CARTESIAN_POINT('Ctrl Pts',(0.4505,1.16034898466907,-1.62253437445173));
#35473=CARTESIAN_POINT('Ctrl Pts',(0.492906278395038,1.70074725201027,-1.23607070952126));
#35474=CARTESIAN_POINT('Ctrl Pts',(0.577718835185113,2.35553983219541,0.112669531194497));
#35475=CARTESIAN_POINT('Ctrl Pts',(0.704937670370226,1.17739386665123,2.04593681646151));
#35476=CARTESIAN_POINT('Ctrl Pts',(0.83215650555534,-1.0826777789212,2.09509384907487));
#35477=CARTESIAN_POINT('Ctrl Pts',(0.959375340740452,-2.34828175108393,
0.223899854992633));
#35478=CARTESIAN_POINT('Ctrl Pts',(1.08659417592557,-1.45844239951523,-1.85436485120368));
#35479=CARTESIAN_POINT('Ctrl Pts',(1.21381301111068,0.770409879037013,-2.22951431439528));
#35480=CARTESIAN_POINT('Ctrl Pts',(1.34103184629579,2.2919408322179,-0.558371212421443));
#35481=CARTESIAN_POINT('Ctrl Pts',(1.4682506814809,1.70949751469815,1.62557712993974));
#35482=CARTESIAN_POINT('Ctrl Pts',(1.59546951666602,-0.442297203023523,
2.3171221778282));
#35483=CARTESIAN_POINT('Ctrl Pts',(1.72268835185113,-2.18804880922234,0.881593520683224));
#35484=CARTESIAN_POINT('Ctrl Pts',(1.84990718703625,-1.92516390965116,-1.36327433887379));
#35485=CARTESIAN_POINT('Ctrl Pts',(1.97712602222136,0.105037018421004,-2.35663178238676));
#35486=CARTESIAN_POINT('Ctrl Pts',(2.10434485740647,2.03881110186596,-1.18659451627925));
#35487=CARTESIAN_POINT('Ctrl Pts',(2.23156369259159,2.1009456770111,1.07274787999985));
#35488=CARTESIAN_POINT('Ctrl Pts',(2.3587825277767,0.234396303221342,2.34729964601711));
#35489=CARTESIAN_POINT('Ctrl Pts',(2.48600136296182,-1.84732607329058,1.46701483016872));
#35490=CARTESIAN_POINT('Ctrl Pts',(2.61322019814693,-2.23319933845391,-0.759995866294124));
#35491=CARTESIAN_POINT('Ctrl Pts',(2.74043903333204,-0.568966582236417,
-2.28933216365562));
#35492=CARTESIAN_POINT('Ctrl Pts',(2.86765786851715,1.61755256653611,-1.71703398256359));
#35493=CARTESIAN_POINT('Ctrl Pts',(2.99487670370227,2.31920284136536,0.43148689290074));
#35494=CARTESIAN_POINT('Ctrl Pts',(3.12209553888738,0.891705714445654,2.18394874208935));
#35495=CARTESIAN_POINT('Ctrl Pts',(3.24931437407249,-1.35418260005473,1.93143856892221));
#35496=CARTESIAN_POINT('Ctrl Pts',(3.37653320925761,-2.35730644925339,-0.0939656234575078));
#35497=CARTESIAN_POINT('Ctrl Pts',(3.50375204444272,-1.19567276206334,-2.03345149280708));
#35498=CARTESIAN_POINT('Ctrl Pts',(3.63097087962784,1.06218487084523,-2.10555757687806));
#35499=CARTESIAN_POINT('Ctrl Pts',(3.75818971481294,2.34767634475008,-0.24602754821659));
#35500=CARTESIAN_POINT('Ctrl Pts',(3.88540854999806,1.47255700028443,1.84196585343814));
#35501=CARTESIAN_POINT('Ctrl Pts',(3.97022110678813,-0.00392161485078923,
2.10247393208426));
#35502=CARTESIAN_POINT('Ctrl Pts',(4.01262738518317,-0.633855508764068,
1.89136320058032));
#35503=CARTESIAN_POINT('Ctrl Pts',(3.7495,-0.778675485261984,2.32349192782157));
#35504=CARTESIAN_POINT('Ctrl Pts',(3.70709372160496,-0.00481760480854909,
2.58283613012782));
#35505=CARTESIAN_POINT('Ctrl Pts',(3.66468744320993,0.902090741196932,2.42282233222775));
#35506=CARTESIAN_POINT('Ctrl Pts',(3.62228116481489,1.53472191663215,1.91530757258047));
#35507=CARTESIAN_POINT('Ctrl Pts',(3.57987488641985,2.16735309206736,1.4077928129332));
#35508=CARTESIAN_POINT('Ctrl Pts',(3.53746860802481,2.5257070969323,0.552777091538723));
#35509=CARTESIAN_POINT('Ctrl Pts',(3.49506232962977,2.44168513067164,-0.255461715829768));
#35510=CARTESIAN_POINT('Ctrl Pts',(3.45265605123473,2.35766316441098,-1.06370052319826));
#35511=CARTESIAN_POINT('Ctrl Pts',(3.4102497728397,1.8312652270247,-1.82516241654077));
#35512=CARTESIAN_POINT('Ctrl Pts',(3.36784349444466,1.10577941123774,-2.19112994599049));
#35513=CARTESIAN_POINT('Ctrl Pts',(3.32543721604962,0.380293595450769,-2.55709747544022));
#35514=CARTESIAN_POINT('Ctrl Pts',(3.28303093765459,-0.544280098736887,
-2.52757064099715));
#35515=CARTESIAN_POINT('Ctrl Pts',(3.24062465925955,-1.24440655400711,-2.11570565525482));
#35516=CARTESIAN_POINT('Ctrl Pts',(3.19821838086451,-1.94453300927732,-1.70384066951249));
#35517=CARTESIAN_POINT('Ctrl Pts',(3.15581210246947,-2.42021222563011,-0.909637532470912));
#35518=CARTESIAN_POINT('Ctrl Pts',(3.11340582407443,-2.45266644779647,-0.0978429804161414));
#35519=CARTESIAN_POINT('Ctrl Pts',(3.11171304812031,-2.45396195706944,-0.0654377246516965));
#35520=CARTESIAN_POINT('Ctrl Pts',(3.11002027216618,-2.45455120914745,-0.0330044378339819));
#35521=CARTESIAN_POINT('Ctrl Pts',(3.10832749621205,-2.45444621147543,-0.000567327939743623));
#35522=CARTESIAN_POINT('Origin',(4.,0.,1.44337567297406));
#35523=CARTESIAN_POINT('',(4.,8.83812698937422E-17,1.44337567297406));
#35524=CARTESIAN_POINT('',(4.,1.25,0.721687836487032));
#35525=CARTESIAN_POINT('',(4.,0.3125,1.26295371385231));
#35526=CARTESIAN_POINT('',(1.8,1.38777878078145E-16,1.44337567297406));
#35527=CARTESIAN_POINT('',(4.,8.83812698937422E-17,1.44337567297406));
#35528=CARTESIAN_POINT('',(1.8,1.25,0.721687836487032));
#35529=CARTESIAN_POINT('',(1.8,1.25,0.721687836487032));
#35530=CARTESIAN_POINT('',(4.,1.25,0.721687836487032));
#35531=CARTESIAN_POINT('Origin',(4.,-1.25,0.721687836487032));
#35532=CARTESIAN_POINT('',(4.,-1.25,0.721687836487032));
#35533=CARTESIAN_POINT('',(4.,-0.9375,0.90210979560879));
#35534=CARTESIAN_POINT('',(1.8,-1.25,0.721687836487032));
#35535=CARTESIAN_POINT('',(4.,-1.25,0.721687836487032));
#35536=CARTESIAN_POINT('',(1.8,8.83812698937422E-17,1.44337567297406));
#35537=CARTESIAN_POINT('Origin',(4.,-1.25,-0.721687836487032));
#35538=CARTESIAN_POINT('',(4.,-1.25,-0.721687836487032));
#35539=CARTESIAN_POINT('',(4.,-1.25,-0.360843918243516));
#35540=CARTESIAN_POINT('',(1.8,-1.25,-0.721687836487032));
#35541=CARTESIAN_POINT('',(4.,-1.25,-0.721687836487032));
#35542=CARTESIAN_POINT('',(1.8,-1.25,0.721687836487032));
#35543=CARTESIAN_POINT('Origin',(4.,-2.77555756156289E-16,-1.44337567297406));
#35544=CARTESIAN_POINT('',(4.,-2.65143809681227E-16,-1.44337567297406));
#35545=CARTESIAN_POINT('',(4.,-0.3125,-1.26295371385231));
#35546=CARTESIAN_POINT('',(1.8,-2.77555756156289E-16,-1.44337567297406));
#35547=CARTESIAN_POINT('',(4.,-2.65143809681227E-16,-1.44337567297406));
#35548=CARTESIAN_POINT('',(1.8,-1.25,-0.721687836487032));
#35549=CARTESIAN_POINT('Origin',(4.,1.25,-0.721687836487033));
#35550=CARTESIAN_POINT('',(4.,1.25,-0.721687836487033));
#35551=CARTESIAN_POINT('',(4.,0.9375,-0.902109795608791));
#35552=CARTESIAN_POINT('',(1.8,1.25,-0.721687836487033));
#35553=CARTESIAN_POINT('',(4.,1.25,-0.721687836487033));
#35554=CARTESIAN_POINT('',(1.8,-2.65143809681227E-16,-1.44337567297406));
#35555=CARTESIAN_POINT('Origin',(4.,1.25,0.721687836487032));
#35556=CARTESIAN_POINT('',(4.,1.25,0.360843918243516));
#35557=CARTESIAN_POINT('',(1.8,1.25,-0.721687836487033));
#35558=CARTESIAN_POINT('Origin',(1.8,0.,0.));
#35559=CARTESIAN_POINT('Origin',(0.,2.,0.));
#35560=CARTESIAN_POINT('',(6.93889390390723E-17,-2.,-2.44929359829471E-16));
#35561=CARTESIAN_POINT('Origin',(0.,0.,0.));
#35562=CARTESIAN_POINT('Origin',(0.25,0.,0.));
#35563=CARTESIAN_POINT('',(0.25,-2.25,-2.75545529808154E-16));
#35564=CARTESIAN_POINT('Origin',(2.1,0.,0.));
#35565=CARTESIAN_POINT('Origin',(3.7495,0.,0.));
#35566=CARTESIAN_POINT('Origin',(3.85,0.,0.));
#35567=CARTESIAN_POINT('',(4.,-2.2,-2.69422295812418E-16));
#35568=CARTESIAN_POINT('Origin',(4.,0.,0.));
#35569=CARTESIAN_POINT('',(3.85,-2.35,-2.87791997799628E-16));
#35570=CARTESIAN_POINT('Origin',(4.,0.,0.));
#38512=UNCERTAINTY_MEASURE_WITH_UNIT(LENGTH_MEASURE(0.01),#38529,
'DISTANCE_ACCURACY_VALUE',
'Maximum model space distance between geometric entities at asserted c
onnectivities');
#38514=UNCERTAINTY_MEASURE_WITH_UNIT(LENGTH_MEASURE(0.01),#38529,
'DISTANCE_ACCURACY_VALUE',
'Maximum model space distance between geometric entities at asserted c
onnectivities');
#38526=(
GEOMETRIC_REPRESENTATION_CONTEXT(3)
GLOBAL_UNCERTAINTY_ASSIGNED_CONTEXT((#38512))
GLOBAL_UNIT_ASSIGNED_CONTEXT((#38529,#38531,#38532))
REPRESENTATION_CONTEXT('','3D')
);
#38528=(
GEOMETRIC_REPRESENTATION_CONTEXT(3)
GLOBAL_UNCERTAINTY_ASSIGNED_CONTEXT((#38514))
GLOBAL_UNIT_ASSIGNED_CONTEXT((#38529,#38531,#38532))
REPRESENTATION_CONTEXT('','3D')
);
#38529=(
LENGTH_UNIT()
NAMED_UNIT(*)
SI_UNIT(.MILLI.,.METRE.)
);
#38531=(
NAMED_UNIT(*)
PLANE_ANGLE_UNIT()
SI_UNIT($,.RADIAN.)
);
#38532=(
NAMED_UNIT(*)
SI_UNIT($,.STERADIAN.)
SOLID_ANGLE_UNIT()
);
#38544=SHAPE_DEFINITION_REPRESENTATION(#38557,#38586);
#38557=PRODUCT_DEFINITION_SHAPE('',$,#38600);
#38586=SHAPE_REPRESENTATION('',(#18774),#38526);
#38588=PRODUCT_DEFINITION_CONTEXT('part definition',#38629,'design');
#38600=PRODUCT_DEFINITION('2026-10-20-13-39-11-796',
'11_ISO_4026_Set_Screw_M5x4',#38613,#38588);
#38613=PRODUCT_DEFINITION_FORMATION('',$,#38642);
#38629=APPLICATION_CONTEXT(
'Core Data for Automotive Mechanical Design Process');
#38630=PRODUCT_CONTEXT('part definition',#38629,'mechanical');
#38642=PRODUCT('2026-10-20-13-39-11-796','11_ISO_4026_Set_Screw_M5x4',$,
(#38630));
#38707=COLOUR_RGB('Black',0.12,0.14,0.17);
#38708=FILL_AREA_STYLE_COLOUR('',#38707);
#38709=FILL_AREA_STYLE('',(#38708));
#38710=SURFACE_STYLE_FILL_AREA(#38709);
#38711=SURFACE_SIDE_STYLE('',(#38710));
#38712=SURFACE_STYLE_USAGE(.BOTH.,#38711);
#38713=PRESENTATION_STYLE_ASSIGNMENT((#38712));
ENDSEC;
END-ISO-10303-21;
